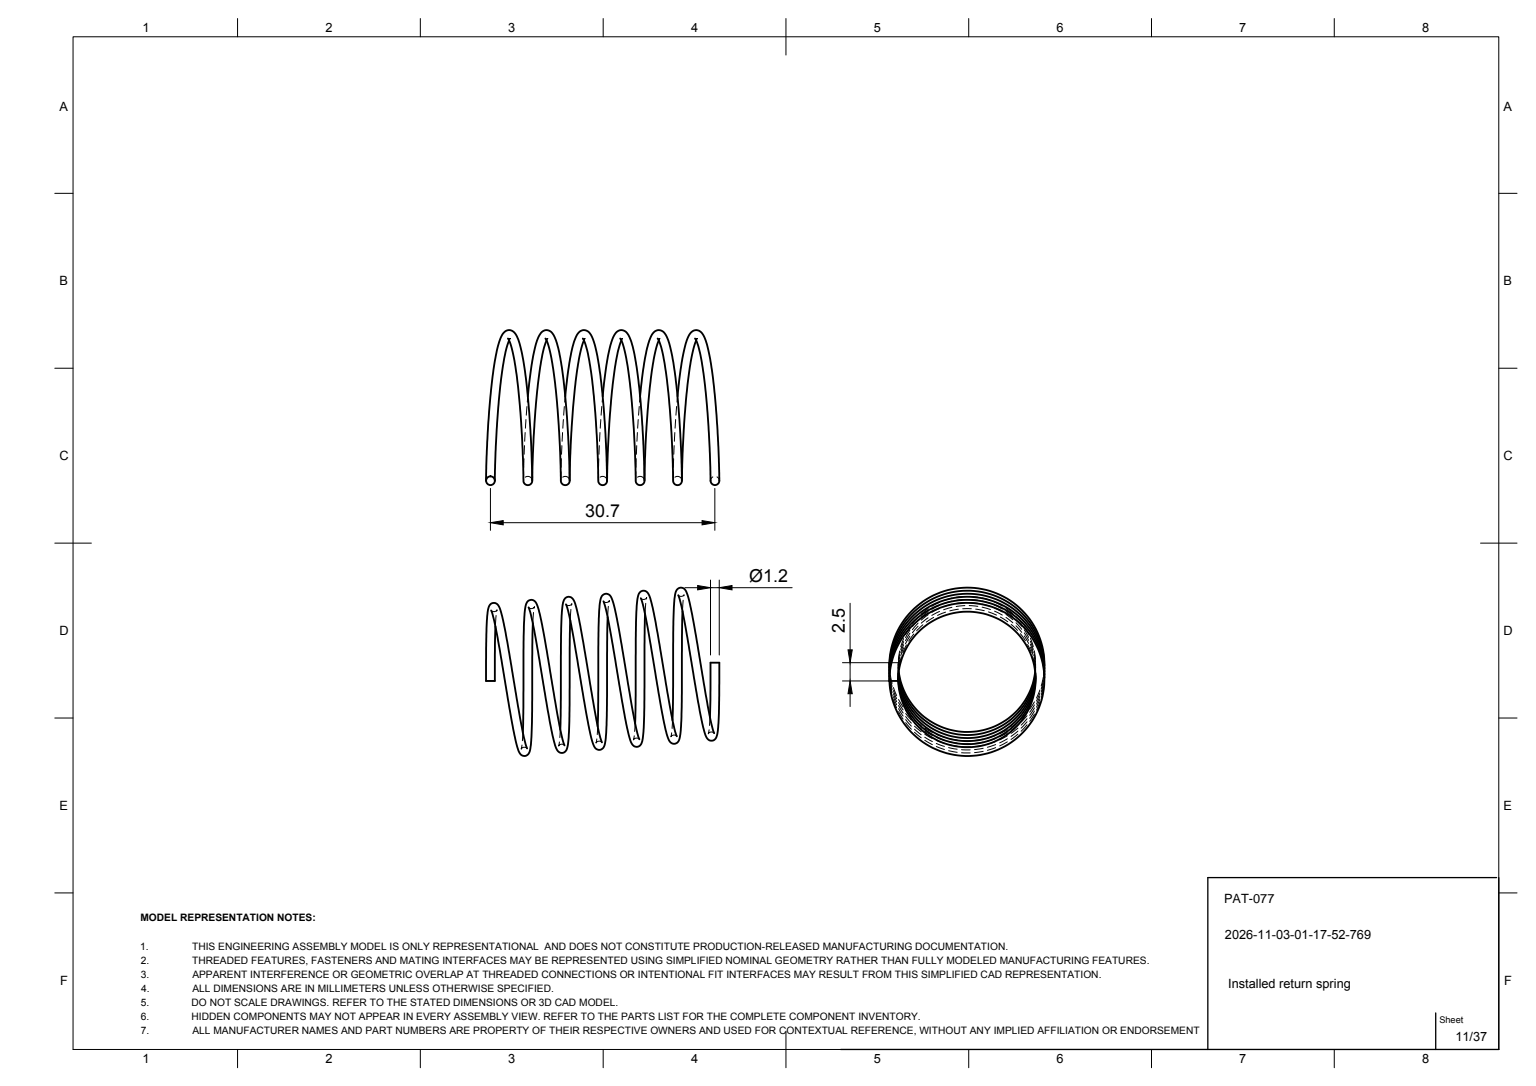
ISO-10303-21;
HEADER;
/* Generated by software containing ST-Developer
 * from STEP Tools, Inc. (www.steptools.com) 
 */

FILE_DESCRIPTION(
/* description */ ('Pallet stop with pneumatic fitting'),
/* implementation_level */ '2;1');

FILE_NAME(
/* name */ 'Installed return spring.step',
/* time_stamp */ '2026-10-27T10:51:41-07:00',
/* author */ (''),
/* organization */ (''),
/* preprocessor_version */ 'ST-DEVELOPER v20.2',
/* originating_system */ 'Autodesk Translation Framework v15.17.0.0',
/* authorisation */ '');

FILE_SCHEMA (('AUTOMOTIVE_DESIGN { 1 0 10303 214 3 1 1 }'));
ENDSEC;

DATA;
#10=MECHANICAL_DESIGN_GEOMETRIC_PRESENTATION_REPRESENTATION('',(#363),#10265);
#280=B_SPLINE_CURVE_WITH_KNOTS('',3,(#8824,#8825,#8826,#8827,#8828,#8829,
#8830,#8831,#8832,#8833,#8834,#8835,#8836,#8837,#8838,#8839,#8840,#8841,
#8842,#8843,#8844,#8845,#8846,#8847,#8848,#8849,#8850,#8851,#8852,#8853,
#8854,#8855,#8856,#8857,#8858,#8859,#8860,#8861,#8862,#8863,#8864,#8865,
#8866,#8867,#8868,#8869,#8870,#8871,#8872,#8873,#8874,#8875,#8876,#8877,
#8878,#8879,#8880,#8881,#8882,#8883,#8884,#8885,#8886,#8887,#8888,#8889,
#8890,#8891,#8892,#8893,#8894,#8895,#8896,#8897,#8898,#8899),
 .UNSPECIFIED.,.F.,.F.,(4,1,1,1,1,1,1,1,1,1,1,1,1,1,1,1,1,1,1,1,1,1,1,1,
1,1,1,1,1,1,1,1,1,1,1,1,1,1,1,1,1,1,1,1,1,1,1,1,1,1,1,1,1,1,1,1,1,1,1,1,
1,1,1,1,1,1,1,1,1,1,1,1,1,4),(0.,0.0178571428571429,0.0357142857142857,
0.0535714285714286,0.0714285714285714,0.0892857142857143,0.107142857142857,
0.125,0.127232142857143,0.129464285714286,0.133928571428571,0.138392857142857,
0.142857142857143,0.158730158730159,0.174603174603175,0.19047619047619,
0.202380952380952,0.214285714285714,0.226190476190476,0.238095238095238,
0.25,0.261904761904762,0.267857142857143,0.273809523809524,0.285714285714286,
0.297619047619048,0.30952380952381,0.321428571428571,0.333333333333333,
0.349206349206349,0.365079365079365,0.373015873015873,0.380952380952381,
0.396825396825397,0.412698412698413,0.428571428571429,0.446428571428571,
0.464285714285714,0.476190476190476,0.488095238095238,0.5,0.517857142857143,
0.535714285714286,0.553571428571429,0.571428571428571,0.589285714285714,
0.607142857142857,0.625,0.642857142857143,0.651785714285714,0.660714285714286,
0.678571428571428,0.696428571428571,0.714285714285714,0.726190476190476,
0.738095238095238,0.75,0.761904761904762,0.773809523809524,0.785714285714286,
0.797619047619047,0.809523809523809,0.821428571428571,0.833333333333333,
0.845238095238095,0.857142857142857,0.875,0.892857142857143,0.910714285714286,
0.928571428571429,0.946428571428571,0.964285714285714,0.982142857142857,
1.),.UNSPECIFIED.);
#292=B_SPLINE_SURFACE_WITH_KNOTS('',3,3,((#8061,#8062,#8063,#8064,#8065,
#8066,#8067,#8068,#8069,#8070,#8071,#8072,#8073,#8074,#8075,#8076,#8077,
#8078,#8079,#8080,#8081,#8082,#8083,#8084,#8085,#8086,#8087,#8088,#8089,
#8090,#8091,#8092,#8093,#8094,#8095,#8096,#8097,#8098,#8099,#8100,#8101,
#8102,#8103,#8104,#8105,#8106,#8107,#8108,#8109,#8110,#8111,#8112,#8113,
#8114,#8115,#8116,#8117,#8118,#8119,#8120,#8121,#8122,#8123,#8124,#8125,
#8126,#8127,#8128,#8129,#8130,#8131,#8132,#8133,#8134,#8135,#8136),(#8137,
#8138,#8139,#8140,#8141,#8142,#8143,#8144,#8145,#8146,#8147,#8148,#8149,
#8150,#8151,#8152,#8153,#8154,#8155,#8156,#8157,#8158,#8159,#8160,#8161,
#8162,#8163,#8164,#8165,#8166,#8167,#8168,#8169,#8170,#8171,#8172,#8173,
#8174,#8175,#8176,#8177,#8178,#8179,#8180,#8181,#8182,#8183,#8184,#8185,
#8186,#8187,#8188,#8189,#8190,#8191,#8192,#8193,#8194,#8195,#8196,#8197,
#8198,#8199,#8200,#8201,#8202,#8203,#8204,#8205,#8206,#8207,#8208,#8209,
#8210,#8211,#8212),(#8213,#8214,#8215,#8216,#8217,#8218,#8219,#8220,#8221,
#8222,#8223,#8224,#8225,#8226,#8227,#8228,#8229,#8230,#8231,#8232,#8233,
#8234,#8235,#8236,#8237,#8238,#8239,#8240,#8241,#8242,#8243,#8244,#8245,
#8246,#8247,#8248,#8249,#8250,#8251,#8252,#8253,#8254,#8255,#8256,#8257,
#8258,#8259,#8260,#8261,#8262,#8263,#8264,#8265,#8266,#8267,#8268,#8269,
#8270,#8271,#8272,#8273,#8274,#8275,#8276,#8277,#8278,#8279,#8280,#8281,
#8282,#8283,#8284,#8285,#8286,#8287,#8288),(#8289,#8290,#8291,#8292,#8293,
#8294,#8295,#8296,#8297,#8298,#8299,#8300,#8301,#8302,#8303,#8304,#8305,
#8306,#8307,#8308,#8309,#8310,#8311,#8312,#8313,#8314,#8315,#8316,#8317,
#8318,#8319,#8320,#8321,#8322,#8323,#8324,#8325,#8326,#8327,#8328,#8329,
#8330,#8331,#8332,#8333,#8334,#8335,#8336,#8337,#8338,#8339,#8340,#8341,
#8342,#8343,#8344,#8345,#8346,#8347,#8348,#8349,#8350,#8351,#8352,#8353,
#8354,#8355,#8356,#8357,#8358,#8359,#8360,#8361,#8362,#8363,#8364),(#8365,
#8366,#8367,#8368,#8369,#8370,#8371,#8372,#8373,#8374,#8375,#8376,#8377,
#8378,#8379,#8380,#8381,#8382,#8383,#8384,#8385,#8386,#8387,#8388,#8389,
#8390,#8391,#8392,#8393,#8394,#8395,#8396,#8397,#8398,#8399,#8400,#8401,
#8402,#8403,#8404,#8405,#8406,#8407,#8408,#8409,#8410,#8411,#8412,#8413,
#8414,#8415,#8416,#8417,#8418,#8419,#8420,#8421,#8422,#8423,#8424,#8425,
#8426,#8427,#8428,#8429,#8430,#8431,#8432,#8433,#8434,#8435,#8436,#8437,
#8438,#8439,#8440),(#8441,#8442,#8443,#8444,#8445,#8446,#8447,#8448,#8449,
#8450,#8451,#8452,#8453,#8454,#8455,#8456,#8457,#8458,#8459,#8460,#8461,
#8462,#8463,#8464,#8465,#8466,#8467,#8468,#8469,#8470,#8471,#8472,#8473,
#8474,#8475,#8476,#8477,#8478,#8479,#8480,#8481,#8482,#8483,#8484,#8485,
#8486,#8487,#8488,#8489,#8490,#8491,#8492,#8493,#8494,#8495,#8496,#8497,
#8498,#8499,#8500,#8501,#8502,#8503,#8504,#8505,#8506,#8507,#8508,#8509,
#8510,#8511,#8512,#8513,#8514,#8515,#8516),(#8517,#8518,#8519,#8520,#8521,
#8522,#8523,#8524,#8525,#8526,#8527,#8528,#8529,#8530,#8531,#8532,#8533,
#8534,#8535,#8536,#8537,#8538,#8539,#8540,#8541,#8542,#8543,#8544,#8545,
#8546,#8547,#8548,#8549,#8550,#8551,#8552,#8553,#8554,#8555,#8556,#8557,
#8558,#8559,#8560,#8561,#8562,#8563,#8564,#8565,#8566,#8567,#8568,#8569,
#8570,#8571,#8572,#8573,#8574,#8575,#8576,#8577,#8578,#8579,#8580,#8581,
#8582,#8583,#8584,#8585,#8586,#8587,#8588,#8589,#8590,#8591,#8592),(#8593,
#8594,#8595,#8596,#8597,#8598,#8599,#8600,#8601,#8602,#8603,#8604,#8605,
#8606,#8607,#8608,#8609,#8610,#8611,#8612,#8613,#8614,#8615,#8616,#8617,
#8618,#8619,#8620,#8621,#8622,#8623,#8624,#8625,#8626,#8627,#8628,#8629,
#8630,#8631,#8632,#8633,#8634,#8635,#8636,#8637,#8638,#8639,#8640,#8641,
#8642,#8643,#8644,#8645,#8646,#8647,#8648,#8649,#8650,#8651,#8652,#8653,
#8654,#8655,#8656,#8657,#8658,#8659,#8660,#8661,#8662,#8663,#8664,#8665,
#8666,#8667,#8668),(#8669,#8670,#8671,#8672,#8673,#8674,#8675,#8676,#8677,
#8678,#8679,#8680,#8681,#8682,#8683,#8684,#8685,#8686,#8687,#8688,#8689,
#8690,#8691,#8692,#8693,#8694,#8695,#8696,#8697,#8698,#8699,#8700,#8701,
#8702,#8703,#8704,#8705,#8706,#8707,#8708,#8709,#8710,#8711,#8712,#8713,
#8714,#8715,#8716,#8717,#8718,#8719,#8720,#8721,#8722,#8723,#8724,#8725,
#8726,#8727,#8728,#8729,#8730,#8731,#8732,#8733,#8734,#8735,#8736,#8737,
#8738,#8739,#8740,#8741,#8742,#8743,#8744),(#8745,#8746,#8747,#8748,#8749,
#8750,#8751,#8752,#8753,#8754,#8755,#8756,#8757,#8758,#8759,#8760,#8761,
#8762,#8763,#8764,#8765,#8766,#8767,#8768,#8769,#8770,#8771,#8772,#8773,
#8774,#8775,#8776,#8777,#8778,#8779,#8780,#8781,#8782,#8783,#8784,#8785,
#8786,#8787,#8788,#8789,#8790,#8791,#8792,#8793,#8794,#8795,#8796,#8797,
#8798,#8799,#8800,#8801,#8802,#8803,#8804,#8805,#8806,#8807,#8808,#8809,
#8810,#8811,#8812,#8813,#8814,#8815,#8816,#8817,#8818,#8819,#8820)),
 .UNSPECIFIED.,.T.,.F.,.F.,(4,1,1,1,1,1,1,4),(4,1,1,1,1,1,1,1,1,1,1,1,1,
1,1,1,1,1,1,1,1,1,1,1,1,1,1,1,1,1,1,1,1,1,1,1,1,1,1,1,1,1,1,1,1,1,1,1,1,
1,1,1,1,1,1,1,1,1,1,1,1,1,1,1,1,1,1,1,1,1,1,1,1,4),(-3.14159265358979,-2.24399475256414,
-1.34639685153848,-0.448798950512828,0.448798950512828,1.34639685153848,
2.24399475256414,3.14159265358979),(0.,0.0178571428571429,0.0357142857142857,
0.0535714285714286,0.0714285714285714,0.0892857142857143,0.107142857142857,
0.125,0.127232142857143,0.129464285714286,0.133928571428571,0.138392857142857,
0.142857142857143,0.158730158730159,0.174603174603175,0.19047619047619,
0.202380952380952,0.214285714285714,0.226190476190476,0.238095238095238,
0.25,0.261904761904762,0.267857142857143,0.273809523809524,0.285714285714286,
0.297619047619048,0.30952380952381,0.321428571428571,0.333333333333333,
0.349206349206349,0.365079365079365,0.373015873015873,0.380952380952381,
0.396825396825397,0.412698412698413,0.428571428571429,0.446428571428571,
0.464285714285714,0.476190476190476,0.488095238095238,0.5,0.517857142857143,
0.535714285714286,0.553571428571429,0.571428571428571,0.589285714285714,
0.607142857142857,0.625,0.642857142857143,0.651785714285714,0.660714285714286,
0.678571428571428,0.696428571428571,0.714285714285714,0.726190476190476,
0.738095238095238,0.75,0.761904761904762,0.773809523809524,0.785714285714286,
0.797619047619047,0.809523809523809,0.821428571428571,0.833333333333333,
0.845238095238095,0.857142857142857,0.875,0.892857142857143,0.910714285714286,
0.928571428571429,0.946428571428571,0.964285714285714,0.982142857142857,
1.),.UNSPECIFIED.);
#299=SHAPE_REPRESENTATION_RELATIONSHIP('SRR','None',#10412,#331);
#331=ADVANCED_BREP_SHAPE_REPRESENTATION('',(#395),#10236);
#363=STYLED_ITEM('',(#10655),#395);
#395=MANIFOLD_SOLID_BREP('Body1',#5051);
#587=PLANE('',#5581);
#588=PLANE('',#5582);
#810=FACE_OUTER_BOUND('',#1170,.T.);
#811=FACE_OUTER_BOUND('',#1171,.T.);
#812=FACE_OUTER_BOUND('',#1172,.T.);
#1170=EDGE_LOOP('',(#3698,#3699,#3700,#3701));
#1171=EDGE_LOOP('',(#3702));
#1172=EDGE_LOOP('',(#3703));
#2224=CIRCLE('',#5579,0.06);
#2225=CIRCLE('',#5580,0.06);
#2503=VERTEX_POINT('',#8821);
#2504=VERTEX_POINT('',#8823);
#2948=EDGE_CURVE('',#2503,#2503,#2224,.T.);
#2949=EDGE_CURVE('',#2503,#2504,#280,.T.);
#2950=EDGE_CURVE('',#2504,#2504,#2225,.T.);
#3698=ORIENTED_EDGE('',*,*,#2948,.T.);
#3699=ORIENTED_EDGE('',*,*,#2949,.T.);
#3700=ORIENTED_EDGE('',*,*,#2950,.F.);
#3701=ORIENTED_EDGE('',*,*,#2949,.F.);
#3702=ORIENTED_EDGE('',*,*,#2950,.T.);
#3703=ORIENTED_EDGE('',*,*,#2948,.F.);
#4805=ADVANCED_FACE('',(#810),#292,.T.);
#4806=ADVANCED_FACE('',(#811),#587,.T.);
#4807=ADVANCED_FACE('',(#812),#588,.F.);
#5051=CLOSED_SHELL('',(#4805,#4806,#4807));
#5578=AXIS2_PLACEMENT_3D('',#8060,#6461,#6462);
#5579=AXIS2_PLACEMENT_3D('',#8822,#6463,#6464);
#5580=AXIS2_PLACEMENT_3D('',#8900,#6465,#6466);
#5581=AXIS2_PLACEMENT_3D('',#8901,#6467,#6468);
#5582=AXIS2_PLACEMENT_3D('',#8902,#6469,#6470);
#6461=DIRECTION('axis',(0.,0.,1.));
#6462=DIRECTION('refdir',(1.,0.,0.));
#6463=DIRECTION('center_axis',(-0.000134470403067858,0.996698884077706,
0.0811869225674069));
#6464=DIRECTION('ref_axis',(1.09533965337888E-5,-0.0811869218285139,0.996698893148795));
#6465=DIRECTION('center_axis',(0.000134470245157523,0.9966988840305,0.0811869231471977));
#6466=DIRECTION('ref_axis',(-0.0717698662269105,0.0809871795599261,-0.994127840395137));
#6467=DIRECTION('center_axis',(0.000134470245157523,0.9966988840305,0.0811869231471977));
#6468=DIRECTION('ref_axis',(-0.0717698662269105,0.0809871795599261,-0.994127840395137));
#6469=DIRECTION('center_axis',(-0.000134470403067858,0.996698884077706,
0.0811869225674069));
#6470=DIRECTION('ref_axis',(1.09533965337888E-5,-0.081186921828514,0.996698893148795));
#8060=CARTESIAN_POINT('',(0.,0.,0.));
#8061=CARTESIAN_POINT('Ctrl Pts',(0.999999342796208,0.0048712153097108,
8.80019806641107));
#8062=CARTESIAN_POINT('Ctrl Pts',(0.99996896462742,0.230035163961994,8.81853897995701));
#8063=CARTESIAN_POINT('Ctrl Pts',(0.843216945008081,0.678245689353448,8.85526000727444));
#8064=CARTESIAN_POINT('Ctrl Pts',(0.23714388778331,1.05999084182087,8.91053070559157));
#8065=CARTESIAN_POINT('Ctrl Pts',(-0.476746387578999,0.979670338171269,
8.96597705173729));
#8066=CARTESIAN_POINT('Ctrl Pts',(-0.98657616663209,0.470389879273211,9.0216024298575));
#8067=CARTESIAN_POINT('Ctrl Pts',(-1.06798165663575,-0.248000588468906,
9.07740270249169));
#8068=CARTESIAN_POINT('Ctrl Pts',(-0.682243081073035,-0.862304425765768,
9.1333764236107));
#8069=CARTESIAN_POINT('Ctrl Pts',(-0.196330490445415,-1.03251494397982,
9.17314484390509));
#8070=CARTESIAN_POINT('Ctrl Pts',(0.0904960552365201,-1.02015022040365,
9.19657718102618));
#8071=CARTESIAN_POINT('Ctrl Pts',(0.204441911777542,-1.00572651008441,9.20595357869542));
#8072=CARTESIAN_POINT('Ctrl Pts',(0.343951015893895,-0.96975630344906,9.21768054548145));
#8073=CARTESIAN_POINT('Ctrl Pts',(0.501773879908335,-0.899045416054097,
9.23176320323934));
#8074=CARTESIAN_POINT('Ctrl Pts',(0.768592409823833,-0.721243151610969,
9.2578611494339));
#8075=CARTESIAN_POINT('Ctrl Pts',(1.04382114359922,-0.318042243912805,9.29602676229045));
#8076=CARTESIAN_POINT('Ctrl Pts',(1.04456490155922,0.326294295864951,9.34634267499162));
#8077=CARTESIAN_POINT('Ctrl Pts',(0.711307557250243,0.815326125223123,9.39257751006242));
#8078=CARTESIAN_POINT('Ctrl Pts',(0.234442425347365,1.04427973165066,9.43469552996756));
#8079=CARTESIAN_POINT('Ctrl Pts',(-0.242097506080382,1.04460426316974,9.47266669612882));
#8080=CARTESIAN_POINT('Ctrl Pts',(-0.672296189994615,0.837312084419627,
9.51070107270169));
#8081=CARTESIAN_POINT('Ctrl Pts',(-0.970493141256397,0.463551157181226,
9.54879683116503));
#8082=CARTESIAN_POINT('Ctrl Pts',(-1.07723336834064,-0.00342794058422688,
9.58695206272228));
#8083=CARTESIAN_POINT('Ctrl Pts',(-0.988260429843343,-0.39307851175747,
9.61879599421848));
#8084=CARTESIAN_POINT('Ctrl Pts',(-0.82093539560644,-0.658946730224756,
9.64429884892662));
#8085=CARTESIAN_POINT('Ctrl Pts',(-0.598840710302034,-0.88141322392247,
9.66981982299092));
#8086=CARTESIAN_POINT('Ctrl Pts',(-0.237756057923814,-1.05547919442497,
9.70175433946707));
#8087=CARTESIAN_POINT('Ctrl Pts',(0.243905786180905,-1.05553040152794,9.74012683420727));
#8088=CARTESIAN_POINT('Ctrl Pts',(0.678604028637572,-0.846341399380819,
9.77854812145871));
#8089=CARTESIAN_POINT('Ctrl Pts',(0.979430107833126,-0.468912235308927,
9.81701586224876));
#8090=CARTESIAN_POINT('Ctrl Pts',(1.09985901046267,0.0548445677701001,9.85980673545165));
#8091=CARTESIAN_POINT('Ctrl Pts',(0.921933505746503,0.631124795915794,9.90693599171239));
#8092=CARTESIAN_POINT('Ctrl Pts',(0.4929126040201,0.973793160670524,9.94983738646297));
#8093=CARTESIAN_POINT('Ctrl Pts',(0.0780904371091028,1.06751269479759,9.98418939216924));
#8094=CARTESIAN_POINT('Ctrl Pts',(-0.346188348797786,1.0365452542535,10.0185609429505));
#8095=CARTESIAN_POINT('Ctrl Pts',(-0.822968443953264,0.76162232341949,10.0615600576428));
#8096=CARTESIAN_POINT('Ctrl Pts',(-1.11011929233597,0.166104281872854,10.1132080400722));
#8097=CARTESIAN_POINT('Ctrl Pts',(-1.0081246602054,-0.515708350877839,10.1670522944212));
#8098=CARTESIAN_POINT('Ctrl Pts',(-0.494775946618556,-1.02970801548153,
10.2230915794475));
#8099=CARTESIAN_POINT('Ctrl Pts',(0.171330015334639,-1.10394798748412,10.2748519542969));
#8100=CARTESIAN_POINT('Ctrl Pts',(0.683814393710209,-0.85633240678914,10.3201591760856));
#8101=CARTESIAN_POINT('Ctrl Pts',(0.987375224349673,-0.475369257557772,
10.3590026286433));
#8102=CARTESIAN_POINT('Ctrl Pts',(1.11501021817459,0.0796008030233853,10.4043267361272));
#8103=CARTESIAN_POINT('Ctrl Pts',(0.894257942603671,0.712772351603783,10.4561304980607));
#8104=CARTESIAN_POINT('Ctrl Pts',(0.254526418580225,1.11465334671006,10.5144063331842));
#8105=CARTESIAN_POINT('Ctrl Pts',(-0.495386650979013,1.03000796421648,10.5726689321936));
#8106=CARTESIAN_POINT('Ctrl Pts',(-1.02902006816757,0.496451864872819,10.6309084916996));
#8107=CARTESIAN_POINT('Ctrl Pts',(-1.11329107431628,-0.25302544687232,10.6891152782939));
#8108=CARTESIAN_POINT('Ctrl Pts',(-0.712411475504087,-0.890954531307481,
10.7472796615617));
#8109=CARTESIAN_POINT('Ctrl Pts',(-0.00144545535703713,-1.13970545531556,
10.8053921361455));
#8110=CARTESIAN_POINT('Ctrl Pts',(0.589562318042014,-0.932130645422847,
10.8537681412278));
#8111=CARTESIAN_POINT('Ctrl Pts',(0.908494555547074,-0.573322783618425,
10.8924337348326));
#8112=CARTESIAN_POINT('Ctrl Pts',(1.0932000203843,-0.130460109720627,10.9310743576345));
#8113=CARTESIAN_POINT('Ctrl Pts',(1.02452819258886,0.49024714203063,10.9793255246093));
#8114=CARTESIAN_POINT('Ctrl Pts',(0.493612168598575,1.02033558321459,11.037138824411));
#8115=CARTESIAN_POINT('Ctrl Pts',(-0.166230575259128,1.09368100121347,11.0884425957329));
#8116=CARTESIAN_POINT('Ctrl Pts',(-0.673140522140151,0.84850197959383,11.1332655331794));
#8117=CARTESIAN_POINT('Ctrl Pts',(-0.973483979429893,0.47222295927322,11.1716363210045));
#8118=CARTESIAN_POINT('Ctrl Pts',(-1.08028898641827,0.00311472479435195,
11.2099559586628));
#8119=CARTESIAN_POINT('Ctrl Pts',(-0.973354083483389,-0.465125791076451,
11.2482222395404));
#8120=CARTESIAN_POINT('Ctrl Pts',(-0.674252322492463,-0.840091585392608,
11.2864330284043));
#8121=CARTESIAN_POINT('Ctrl Pts',(-0.242715089956039,-1.04789098180051,
11.3245862592493));
#8122=CARTESIAN_POINT('Ctrl Pts',(0.23542767696283,-1.04765866302507,11.3626799542613));
#8123=CARTESIAN_POINT('Ctrl Pts',(0.665536159094464,-0.840435751119737,
11.4007121983223));
#8124=CARTESIAN_POINT('Ctrl Pts',(0.962591820228485,-0.467820172164233,
11.4386811727585));
#8125=CARTESIAN_POINT('Ctrl Pts',(1.06846208937938,-0.00379118886353965,
11.47658513569));
#8126=CARTESIAN_POINT('Ctrl Pts',(0.962501175338684,0.458913289962351,11.5144224357756));
#8127=CARTESIAN_POINT('Ctrl Pts',(0.618041205754224,0.892154566858533,11.5584863515166));
#8128=CARTESIAN_POINT('Ctrl Pts',(0.00421838652791971,1.10738146763147,
11.6087289304493));
#8129=CARTESIAN_POINT('Ctrl Pts',(-0.685284502455283,0.86560690604705,11.6650903417562));
#8130=CARTESIAN_POINT('Ctrl Pts',(-1.07219887432344,0.249028474249683,11.7212863124465));
#8131=CARTESIAN_POINT('Ctrl Pts',(-0.990640181337795,-0.472396051339649,
11.7773128627812));
#8132=CARTESIAN_POINT('Ctrl Pts',(-0.478640001005609,-0.983760746265736,
11.8331676524783));
#8133=CARTESIAN_POINT('Ctrl Pts',(0.238202676882345,-1.06445286799178,11.8888462567429));
#8134=CARTESIAN_POINT('Ctrl Pts',(0.846858663881909,-0.681098479204223,
11.9443505326692));
#8135=CARTESIAN_POINT('Ctrl Pts',(1.00427568511571,-0.230977292777482,11.9812290386622));
#8136=CARTESIAN_POINT('Ctrl Pts',(1.00430619197361,-0.004859230773597,11.9996476704237));
#8137=CARTESIAN_POINT('Ctrl Pts',(0.982047384939078,0.00486879330739147,
8.80019806641107));
#8138=CARTESIAN_POINT('Ctrl Pts',(0.982017542571237,0.226061368380877,8.8182154884749));
#8139=CARTESIAN_POINT('Ctrl Pts',(0.828073759479322,0.666265246409587,8.85427793870567));
#8140=CARTESIAN_POINT('Ctrl Pts',(0.232718051648345,1.04130280902705,8.90857206776144));
#8141=CARTESIAN_POINT('Ctrl Pts',(-0.468680551990921,0.962405317361456,
8.96304474127639));
#8142=CARTESIAN_POINT('Ctrl Pts',(-0.969725556632444,0.461952106094082,
9.01770706443454));
#8143=CARTESIAN_POINT('Ctrl Pts',(-1.04978892409544,-0.24421501980538,9.07255473573053));
#8144=CARTESIAN_POINT('Ctrl Pts',(-0.670526282680969,-0.848287475569065,
9.12759197393209));
#8145=CARTESIAN_POINT('Ctrl Pts',(-0.192569344974563,-1.01574821805213,
9.16670672447678));
#8146=CARTESIAN_POINT('Ctrl Pts',(0.0896475808341612,-1.00358230969371,
9.18976208492581));
#8147=CARTESIAN_POINT('Ctrl Pts',(0.201768534269143,-0.989389860609658,
9.19898826062923));
#8148=CARTESIAN_POINT('Ctrl Pts',(0.339053092327797,-0.953994606992962,
9.21052787927458));
#8149=CARTESIAN_POINT('Ctrl Pts',(0.494377601147851,-0.884404812313703,
9.22438724394839));
#8150=CARTESIAN_POINT('Ctrl Pts',(0.757001856405022,-0.709402012144092,
9.25007419376896));
#8151=CARTESIAN_POINT('Ctrl Pts',(1.0279911029959,-0.312481730693998,9.28764301092837));
#8152=CARTESIAN_POINT('Ctrl Pts',(1.02877459893023,0.322165970926696,9.33720097094436));
#8153=CARTESIAN_POINT('Ctrl Pts',(0.700413157880328,0.804092297036147,9.38275776600637));
#8154=CARTESIAN_POINT('Ctrl Pts',(0.230301769583314,1.02983016988876,9.42427724831843));
#8155=CARTESIAN_POINT('Ctrl Pts',(-0.239683635592506,1.03017515445717,9.46172242153018));
#8156=CARTESIAN_POINT('Ctrl Pts',(-0.664163045312016,0.825661502108212,
9.49924891917935));
#8157=CARTESIAN_POINT('Ctrl Pts',(-0.958529939902563,0.456745656141783,
9.53684906905032));
#8158=CARTESIAN_POINT('Ctrl Pts',(-1.06396267414552,-0.00440524776029272,
9.5745255639511));
#8159=CARTESIAN_POINT('Ctrl Pts',(-0.976079979910487,-0.389373735213914,
9.60598297021468));
#8160=CARTESIAN_POINT('Ctrl Pts',(-0.810705582541046,-0.652150929778934,
9.63118793351945));
#8161=CARTESIAN_POINT('Ctrl Pts',(-0.591146716083035,-0.872084267774335,
9.6564168813747));
#8162=CARTESIAN_POINT('Ctrl Pts',(-0.234072078906085,-1.04424533055482,
9.68799397302578));
#8163=CARTESIAN_POINT('Ctrl Pts',(0.242500469223428,-1.04432630242473,9.72595785040098));
#8164=CARTESIAN_POINT('Ctrl Pts',(0.672838065087217,-0.83726980079961,9.7639884443319));
#8165=CARTESIAN_POINT('Ctrl Pts',(0.970815428000762,-0.463458065904377,
9.80208605881035));
#8166=CARTESIAN_POINT('Ctrl Pts',(1.09019540146654,0.0555635056652221,9.84448580287717));
#8167=CARTESIAN_POINT('Ctrl Pts',(0.913813691461406,0.627036825844031,9.89121709087636));
#8168=CARTESIAN_POINT('Ctrl Pts',(0.48811414653708,0.967138669436487,9.93378708715817));
#8169=CARTESIAN_POINT('Ctrl Pts',(0.0762229670049308,1.06020598638962,9.96789328622913));
#8170=CARTESIAN_POINT('Ctrl Pts',(-0.345222042701214,1.0294593023382,10.0020337480872));
#8171=CARTESIAN_POINT('Ctrl Pts',(-0.819095169387929,0.756280403334857,
10.044760955629));
#8172=CARTESIAN_POINT('Ctrl Pts',(-1.10479169712882,0.163970602181336,10.0961315732279));
#8173=CARTESIAN_POINT('Ctrl Pts',(-1.00334187935937,-0.514754332116599,
10.1497258011113));
#8174=CARTESIAN_POINT('Ctrl Pts',(-0.491985150485256,-1.0269135369247,10.2055489936168));
#8175=CARTESIAN_POINT('Ctrl Pts',(0.172230476805367,-1.10104324987106,10.2571555969155));
#8176=CARTESIAN_POINT('Ctrl Pts',(0.6837034079542,-0.853959036612514,10.3023689497361));
#8177=CARTESIAN_POINT('Ctrl Pts',(0.986863059949987,-0.473547176850352,
10.3411560919635));
#8178=CARTESIAN_POINT('Ctrl Pts',(1.11443827396583,0.0809655868366956,10.3864406203787));
#8179=CARTESIAN_POINT('Ctrl Pts',(0.893794220249733,0.714129022372665,10.4382345485064));
#8180=CARTESIAN_POINT('Ctrl Pts',(0.253564991089117,1.11646188695564,10.4965555791176));
#8181=CARTESIAN_POINT('Ctrl Pts',(-0.497710807257122,1.03177486246381,10.5549164707911));
#8182=CARTESIAN_POINT('Ctrl Pts',(-1.03287455412715,0.496850894811073,10.6133080838302));
#8183=CARTESIAN_POINT('Ctrl Pts',(-1.11756500239139,-0.255330318551581,
10.6717198630721));
#8184=CARTESIAN_POINT('Ctrl Pts',(-0.714971732167115,-0.896204048773918,
10.7301410140639));
#8185=CARTESIAN_POINT('Ctrl Pts',(-0.000197744427673544,-1.14640555699347,
10.7885625557949));
#8186=CARTESIAN_POINT('Ctrl Pts',(0.594542321544182,-0.937612040665249,
10.8372358480802));
#8187=CARTESIAN_POINT('Ctrl Pts',(0.915705377171634,-0.576320258708504,
10.8761680572913));
#8188=CARTESIAN_POINT('Ctrl Pts',(1.10178414791373,-0.130204417591924,10.915091761851));
#8189=CARTESIAN_POINT('Ctrl Pts',(1.03265373134923,0.495463186235901,10.9637246794375));
#8190=CARTESIAN_POINT('Ctrl Pts',(0.497145233405868,1.03028230225543,11.0220401925551));
#8191=CARTESIAN_POINT('Ctrl Pts',(-0.169012977210461,1.10441503835764,11.0738304261316));
#8192=CARTESIAN_POINT('Ctrl Pts',(-0.681133539914993,0.85674905407542,11.1191103749823));
#8193=CARTESIAN_POINT('Ctrl Pts',(-0.984721103773031,0.476446874844114,
11.1578900621551));
#8194=CARTESIAN_POINT('Ctrl Pts',(-1.092751156294,0.00206620542347027,11.1966396932756));
#8195=CARTESIAN_POINT('Ctrl Pts',(-0.98459016094734,-0.471660870020862,
11.2353514494943));
#8196=CARTESIAN_POINT('Ctrl Pts',(-0.681864802424284,-0.851204764218623,
11.2740254978417));
#8197=CARTESIAN_POINT('Ctrl Pts',(-0.244894669388729,-1.06164493769735,
11.3126574520722));
#8198=CARTESIAN_POINT('Ctrl Pts',(0.239497914027533,-1.06142946990311,11.3512480535563));
#8199=CARTESIAN_POINT('Ctrl Pts',(0.675410001418759,-0.85143262563631,11.3897909190191));
#8200=CARTESIAN_POINT('Ctrl Pts',(0.97660256231849,-0.47365645262325,11.4282852412925));
#8201=CARTESIAN_POINT('Ctrl Pts',(1.08400003731686,-0.00301072745489087,
11.4667285195545));
#8202=CARTESIAN_POINT('Ctrl Pts',(0.976502876676812,0.466470502386992,11.5051182694331));
#8203=CARTESIAN_POINT('Ctrl Pts',(0.626894863562504,0.906218485725883,11.549841630365));
#8204=CARTESIAN_POINT('Ctrl Pts',(0.00363437595233928,1.12480301808217,
11.600855774006));
#8205=CARTESIAN_POINT('Ctrl Pts',(-0.696824177011358,0.879241198259212,
11.6581097453269));
#8206=CARTESIAN_POINT('Ctrl Pts',(-1.09007389999346,0.25264708501371,11.7152189643452));
#8207=CARTESIAN_POINT('Ctrl Pts',(-1.00719470908938,-0.480789320374471,
11.7721773844949));
#8208=CARTESIAN_POINT('Ctrl Pts',(-0.486528264941766,-1.00085757657432,
11.8289789551926));
#8209=CARTESIAN_POINT('Ctrl Pts',(0.242674951053419,-1.08295512724231,11.8856179806837));
#8210=CARTESIAN_POINT('Ctrl Pts',(0.861972926357441,-0.692938107583723,
11.9420899351664));
#8211=CARTESIAN_POINT('Ctrl Pts',(1.02218081422145,-0.234837326490113,11.9796219395556));
#8212=CARTESIAN_POINT('Ctrl Pts',(1.02221185564686,-0.00475702858911594,
11.9983633184843));
#8213=CARTESIAN_POINT('Ctrl Pts',(0.946251939821601,0.00346790923095878,
8.81733686319961));
#8214=CARTESIAN_POINT('Ctrl Pts',(0.946223170149248,0.216709631387298,8.83470664203795));
#8215=CARTESIAN_POINT('Ctrl Pts',(0.797868558912845,0.640717122048251,8.86944390364538));
#8216=CARTESIAN_POINT('Ctrl Pts',(0.224685675994098,1.00171482448492,8.92171403423268));
#8217=CARTESIAN_POINT('Ctrl Pts',(-0.450094354194183,0.925721174112207,
8.97411924922092));
#8218=CARTESIAN_POINT('Ctrl Pts',(-0.931851520616104,0.444457369493084,
9.02668243919957));
#8219=CARTESIAN_POINT('Ctrl Pts',(-1.00876374936087,-0.234332975359601,
9.07940345376113));
#8220=CARTESIAN_POINT('Ctrl Pts',(-0.644280498352913,-0.814814073429451,
9.132293292668));
#8221=CARTESIAN_POINT('Ctrl Pts',(-0.185030806522485,-0.975710075967432,
9.16987780176979));
#8222=CARTESIAN_POINT('Ctrl Pts',(0.0861306964382634,-0.964020787510786,
9.19203012360292));
#8223=CARTESIAN_POINT('Ctrl Pts',(0.193859203693136,-0.950384199462588,
9.20089488110907));
#8224=CARTESIAN_POINT('Ctrl Pts',(0.325766432724325,-0.916374835785051,
9.21198266561942));
#8225=CARTESIAN_POINT('Ctrl Pts',(0.475008489408351,-0.849509651707339,
9.22529946397773));
#8226=CARTESIAN_POINT('Ctrl Pts',(0.72735253136785,-0.681355419969213,9.2499813528838));
#8227=CARTESIAN_POINT('Ctrl Pts',(0.987759532431315,-0.299937694770344,
9.28608546277695));
#8228=CARTESIAN_POINT('Ctrl Pts',(0.988529254394412,0.31002344397511,9.33371680705976));
#8229=CARTESIAN_POINT('Ctrl Pts',(0.67286673528341,0.773354286803788,9.37751699303838));
#8230=CARTESIAN_POINT('Ctrl Pts',(0.220764282478621,0.990462726141864,9.41744839941452));
#8231=CARTESIAN_POINT('Ctrl Pts',(-0.23137446087799,0.990807495240239,9.45347433529735));
#8232=CARTESIAN_POINT('Ctrl Pts',(-0.639893401702073,0.794007818769354,
9.48958994897445));
#8233=CARTESIAN_POINT('Ctrl Pts',(-0.923327263108843,0.438822435846309,
9.52579447470907));
#8234=CARTESIAN_POINT('Ctrl Pts',(-1.02491137571836,-0.00538407263128216,
9.56208933392858));
#8235=CARTESIAN_POINT('Ctrl Pts',(-0.940232267608687,-0.376417877351174,
9.59241037531266));
#8236=CARTESIAN_POINT('Ctrl Pts',(-0.780786057662726,-0.629783667326523,
9.61671320097693));
#8237=CARTESIAN_POINT('Ctrl Pts',(-0.569033793255791,-0.841902767826415,
9.64104641368153));
#8238=CARTESIAN_POINT('Ctrl Pts',(-0.224489149210013,-1.0080482857871,9.67151952337384));
#8239=CARTESIAN_POINT('Ctrl Pts',(0.235673510791263,-1.00815805640934,9.70817893472068));
#8240=CARTESIAN_POINT('Ctrl Pts',(0.651503567024935,-0.808120949371662,
9.74492970282906));
#8241=CARTESIAN_POINT('Ctrl Pts',(0.939670159494493,-0.446677535335527,
9.78177187806484));
#8242=CARTESIAN_POINT('Ctrl Pts',(1.05523972468657,0.0555890051172364,9.82280879182749));
#8243=CARTESIAN_POINT('Ctrl Pts',(0.884483903066246,0.609188073050605,9.86807884630888));
#8244=CARTESIAN_POINT('Ctrl Pts',(0.471693669376953,0.939087262360839,9.90936701071719));
#8245=CARTESIAN_POINT('Ctrl Pts',(0.0718701946233878,1.02945078127861,9.94247676831493));
#8246=CARTESIAN_POINT('Ctrl Pts',(-0.337475699762535,0.999603452125411,
9.97563909649433));
#8247=CARTESIAN_POINT('Ctrl Pts',(-0.798276925818471,0.734084817620259,
10.0171900420759));
#8248=CARTESIAN_POINT('Ctrl Pts',(-1.0765334634925,0.157487645860965,10.0672053034725));
#8249=CARTESIAN_POINT('Ctrl Pts',(-0.977769536461385,-0.504250043799724,
10.1194626321329));
#8250=CARTESIAN_POINT('Ctrl Pts',(-0.478575291848728,-1.00451835916292,
10.1739816819444));
#8251=CARTESIAN_POINT('Ctrl Pts',(0.171126569807208,-1.07721754138009,10.2244700816925));
#8252=CARTESIAN_POINT('Ctrl Pts',(0.672182788674072,-0.835256219302107,
10.2687619732111));
#8253=CARTESIAN_POINT('Ctrl Pts',(0.969547810320499,-0.462213248235356,
10.3068036909456));
#8254=CARTESIAN_POINT('Ctrl Pts',(1.09489348151214,0.0822563931149444,10.3512740281145));
#8255=CARTESIAN_POINT('Ctrl Pts',(0.878086601000876,0.705028239333339,10.4022206349257));
#8256=CARTESIAN_POINT('Ctrl Pts',(0.247376731962901,1.10167051144662,10.4596936844876));
#8257=CARTESIAN_POINT('Ctrl Pts',(-0.494343825650103,1.01831274777828,10.5173179494214));
#8258=CARTESIAN_POINT('Ctrl Pts',(-1.02389367392556,0.489356402466505,10.5750854103097));
#8259=CARTESIAN_POINT('Ctrl Pts',(-1.1080879323535,-0.256139394666961,10.6329877640774));
#8260=CARTESIAN_POINT('Ctrl Pts',(-0.708467620348485,-0.892752715736136,
10.6910165384584));
#8261=CARTESIAN_POINT('Ctrl Pts',(0.00275806339120792,-1.14199252167361,
10.7491621240617));
#8262=CARTESIAN_POINT('Ctrl Pts',(0.595915072591307,-0.933982364866608,
10.7977073894074));
#8263=CARTESIAN_POINT('Ctrl Pts',(0.916693997947134,-0.573186172446775,
10.8365910184109));
#8264=CARTESIAN_POINT('Ctrl Pts',(1.10275571560074,-0.127229568265828,10.8755054547366));
#8265=CARTESIAN_POINT('Ctrl Pts',(1.03374107847987,0.499230126741185,10.9242044521008));
#8266=CARTESIAN_POINT('Ctrl Pts',(0.496651096330989,1.03602339561547,10.982721896355));
#8267=CARTESIAN_POINT('Ctrl Pts',(-0.173057151953294,1.11077134701646,11.0347972056812));
#8268=CARTESIAN_POINT('Ctrl Pts',(-0.688810280773869,0.861454433490338,
11.0803977479046));
#8269=CARTESIAN_POINT('Ctrl Pts',(-0.994990321540318,0.478015999913525,
11.1195067251792));
#8270=CARTESIAN_POINT('Ctrl Pts',(-1.10413900699883,-0.000930907827253689,
11.1586323799395));
#8271=CARTESIAN_POINT('Ctrl Pts',(-0.994852434030972,-0.479892724154501,
11.1977747838273));
#8272=CARTESIAN_POINT('Ctrl Pts',(-0.688454851688791,-0.864158828181502,
11.2369285531699));
#8273=CARTESIAN_POINT('Ctrl Pts',(-0.245556936433115,-1.07753293814173,
11.2760917573129));
#8274=CARTESIAN_POINT('Ctrl Pts',(0.246044401600366,-1.0773877681717,11.3152583014517));
#8275=CARTESIAN_POINT('Ctrl Pts',(0.689038817571119,-0.864056889518542,
11.3544280678403));
#8276=CARTESIAN_POINT('Ctrl Pts',(0.995533503363568,-0.479743995432174,
11.3935962007367));
#8277=CARTESIAN_POINT('Ctrl Pts',(1.10500493611492,-0.000336441793609564,
11.432759423983));
#8278=CARTESIAN_POINT('Ctrl Pts',(0.995437508199075,0.478484225555593,11.471914533027));
#8279=CARTESIAN_POINT('Ctrl Pts',(0.638543403370204,0.927530552036555,11.5175815981191));
#8280=CARTESIAN_POINT('Ctrl Pts',(0.00131834384992748,1.1512205599446,11.5697498749575));
#8281=CARTESIAN_POINT('Ctrl Pts',(-0.716162033397229,0.899924142153474,
11.6283938640621));
#8282=CARTESIAN_POINT('Ctrl Pts',(-1.11974363778359,0.257254170951805,11.6869825988179));
#8283=CARTESIAN_POINT('Ctrl Pts',(-1.03478697806096,-0.496287761111256,
11.7455056502723));
#8284=CARTESIAN_POINT('Ctrl Pts',(-0.499211397844794,-1.0315157806068,11.8039508889109));
#8285=CARTESIAN_POINT('Ctrl Pts',(0.25207649193241,-1.11624858861966,11.8623120440781));
#8286=CARTESIAN_POINT('Ctrl Pts',(0.891057567372483,-0.71406944827229,11.9205699244295));
#8287=CARTESIAN_POINT('Ctrl Pts',(1.05664899061948,-0.24083687143616,11.9593476619553));
#8288=CARTESIAN_POINT('Ctrl Pts',(1.05668105685756,-0.00316062068079096,
11.9787077754391));
#8289=CARTESIAN_POINT('Ctrl Pts',(0.933110845774544,-0.00124761587970791,
8.87520568466563));
#8290=CARTESIAN_POINT('Ctrl Pts',(0.933082485311987,0.208961030315505,8.89232840182152));
#8291=CARTESIAN_POINT('Ctrl Pts',(0.786770179169481,0.626345163412827,8.92653493659135));
#8292=CARTESIAN_POINT('Ctrl Pts',(0.224133602875593,0.980245228608542,8.97782692366071));
#8293=CARTESIAN_POINT('Ctrl Pts',(-0.435812671372105,0.905573247736591,
9.02908909375654));
#8294=CARTESIAN_POINT('Ctrl Pts',(-0.905278949446739,0.436102668627462,
9.08034196302577));
#8295=CARTESIAN_POINT('Ctrl Pts',(-0.979701853601785,-0.223724459540056,
9.13159318793611));
#8296=CARTESIAN_POINT('Ctrl Pts',(-0.626199332431556,-0.786111248844846,
9.18285439354528));
#8297=CARTESIAN_POINT('Ctrl Pts',(-0.182309307756624,-0.941401852206475,
9.21918157669349));
#8298=CARTESIAN_POINT('Ctrl Pts',(0.0793196104033138,-0.930122621318997,
9.24055595057928));
#8299=CARTESIAN_POINT('Ctrl Pts',(0.183226682424838,-0.916969037284389,
9.24910628913725));
#8300=CARTESIAN_POINT('Ctrl Pts',(0.310391085781095,-0.884178026616486,
9.25979589713383));
#8301=CARTESIAN_POINT('Ctrl Pts',(0.454169054244644,-0.819756142740368,
9.27262568518493));
#8302=CARTESIAN_POINT('Ctrl Pts',(0.697116053142912,-0.657850695056992,
9.29638934987471));
#8303=CARTESIAN_POINT('Ctrl Pts',(0.947351969011777,-0.291063703435681,
9.33110485588488));
#8304=CARTESIAN_POINT('Ctrl Pts',(0.947893979854482,0.294038239775498,9.37679585569485));
#8305=CARTESIAN_POINT('Ctrl Pts',(0.64559614597452,0.737470402080906,9.41872694647258));
#8306=CARTESIAN_POINT('Ctrl Pts',(0.213542771693588,0.944865687214638,9.456887453317));
#8307=CARTESIAN_POINT('Ctrl Pts',(-0.21790942255983,0.945130416632738,9.49126781446859));
#8308=CARTESIAN_POINT('Ctrl Pts',(-0.607175295083612,0.757538118255783,
9.52568490650978));
#8309=CARTESIAN_POINT('Ctrl Pts',(-0.876886139203015,0.419454940311435,
9.5601447217719));
#8310=CARTESIAN_POINT('Ctrl Pts',(-0.973399204055829,-0.00281983355499825,
9.59464850829951));
#8311=CARTESIAN_POINT('Ctrl Pts',(-0.892953621384232,-0.355121345095021,
9.62344157007163));
#8312=CARTESIAN_POINT('Ctrl Pts',(-0.741670531971874,-0.595502068510008,
9.64649995731916));
#8313=CARTESIAN_POINT('Ctrl Pts',(-0.540861334347598,-0.79664831552706,
9.66957548515654));
#8314=CARTESIAN_POINT('Ctrl Pts',(-0.214347909139945,-0.954058224911974,
9.69845416164799));
#8315=CARTESIAN_POINT('Ctrl Pts',(0.221317761541613,-0.954121235060302,
9.73316338989386));
#8316=CARTESIAN_POINT('Ctrl Pts',(0.614674372570484,-0.764854624133257,
9.76793103575109));
#8317=CARTESIAN_POINT('Ctrl Pts',(0.887052993147029,-0.423164929085746,
9.80275900129157));
#8318=CARTESIAN_POINT('Ctrl Pts',(0.996196176963173,0.0513246907769201,
9.8415273466477));
#8319=CARTESIAN_POINT('Ctrl Pts',(0.834948113879409,0.573926065074171,9.88426514494727));
#8320=CARTESIAN_POINT('Ctrl Pts',(0.44547575217633,0.885137394010584,9.92321920683063));
#8321=CARTESIAN_POINT('Ctrl Pts',(0.0684014908627373,0.970356094387837,
9.95444592358018));
#8322=CARTESIAN_POINT('Ctrl Pts',(-0.317575790754665,0.942207118119873,
9.98571530594194));
#8323=CARTESIAN_POINT('Ctrl Pts',(-0.751956369176069,0.691895051315754,
10.0248858146619));
#8324=CARTESIAN_POINT('Ctrl Pts',(-1.01420012669963,0.148454419987656,10.0720248209112));
#8325=CARTESIAN_POINT('Ctrl Pts',(-0.921125606711717,-0.475192219958838,
10.1212746978924));
#8326=CARTESIAN_POINT('Ctrl Pts',(-0.450640791192364,-0.946727050507445,
10.1726608327701));
#8327=CARTESIAN_POINT('Ctrl Pts',(0.161885358038663,-1.0153085919114,10.2202607279042));
#8328=CARTESIAN_POINT('Ctrl Pts',(0.634464325836929,-0.7871254203658,10.2620342877094));
#8329=CARTESIAN_POINT('Ctrl Pts',(0.915044949089008,-0.435171331085412,
10.2979265084477));
#8330=CARTESIAN_POINT('Ctrl Pts',(1.0333921730293,0.0787559345129345,10.3399027505605));
#8331=CARTESIAN_POINT('Ctrl Pts',(0.828697304223945,0.667017539209564,10.3880228606081));
#8332=CARTESIAN_POINT('Ctrl Pts',(0.232467374207285,1.04212743993356,10.4423591262489));
#8333=CARTESIAN_POINT('Ctrl Pts',(-0.469582947467488,0.963374254330498,
10.4968986206485));
#8334=CARTESIAN_POINT('Ctrl Pts',(-0.971549690422633,0.462203568299623,
10.5516426651414));
#8335=CARTESIAN_POINT('Ctrl Pts',(-1.05163594424887,-0.245277711367363,
10.6065920927203));
#8336=CARTESIAN_POINT('Ctrl Pts',(-0.671962136426674,-0.850494803107478,
10.6617469196619));
#8337=CARTESIAN_POINT('Ctrl Pts',(0.00514473529517556,-1.08801203030429,
10.7171069354582));
#8338=CARTESIAN_POINT('Ctrl Pts',(0.571006381985689,-0.889777195779423,
10.7634098332665));
#8339=CARTESIAN_POINT('Ctrl Pts',(0.877482655626295,-0.545130724676744,
10.8005540126445));
#8340=CARTESIAN_POINT('Ctrl Pts',(1.05543893274011,-0.118705473665279,10.8377653530311));
#8341=CARTESIAN_POINT('Ctrl Pts',(0.989557126951709,0.481292167662269,10.8844038712234));
#8342=CARTESIAN_POINT('Ctrl Pts',(0.474249124300982,0.996731925119642,10.9405665516539));
#8343=CARTESIAN_POINT('Ctrl Pts',(-0.170018784224988,1.06889843758203,10.9906607188205));
#8344=CARTESIAN_POINT('Ctrl Pts',(-0.667252349418254,0.828652140244528,
11.0346171254776));
#8345=CARTESIAN_POINT('Ctrl Pts',(-0.962957118749545,0.458476875796659,
11.0723761453514));
#8346=CARTESIAN_POINT('Ctrl Pts',(-1.06861617984619,-0.00474659541608284,
11.1102178529854));
#8347=CARTESIAN_POINT('Ctrl Pts',(-0.962829285747689,-0.468812774742328,
11.1481382421668));
#8348=CARTESIAN_POINT('Ctrl Pts',(-0.66552637265583,-0.841826091853817,
11.1861371971565));
#8349=CARTESIAN_POINT('Ctrl Pts',(-0.234945846970159,-1.0493782184629,11.2242118409212));
#8350=CARTESIAN_POINT('Ctrl Pts',(0.243922228184406,-1.04933364959166,11.2623624755123));
#8351=CARTESIAN_POINT('Ctrl Pts',(0.676275279337915,-0.841241205435662,
11.3005845553303));
#8352=CARTESIAN_POINT('Ctrl Pts',(0.976019367363091,-0.465554703444286,
11.3388772265428));
#8353=CARTESIAN_POINT('Ctrl Pts',(1.08335811630658,0.00404254183906937,
11.3772382701768));
#8354=CARTESIAN_POINT('Ctrl Pts',(0.975916530883124,0.474019295230167,11.4156652984567));
#8355=CARTESIAN_POINT('Ctrl Pts',(0.625055282289429,0.915683137019696,11.4605716003999));
#8356=CARTESIAN_POINT('Ctrl Pts',(-0.00300719915789507,1.13650050171769,
11.5119933522144));
#8357=CARTESIAN_POINT('Ctrl Pts',(-0.712553859124697,0.888397715677925,
11.5699732202525));
#8358=CARTESIAN_POINT('Ctrl Pts',(-1.1131339679836,0.251233314201274,11.6280728566751));
#8359=CARTESIAN_POINT('Ctrl Pts',(-1.02901641656587,-0.498400062976102,
11.6862845413367));
#8360=CARTESIAN_POINT('Ctrl Pts',(-0.494901381262588,-1.03273028842869,
11.7445959726463));
#8361=CARTESIAN_POINT('Ctrl Pts',(0.256963427041344,-1.11790522486644,11.8030028921807));
#8362=CARTESIAN_POINT('Ctrl Pts',(0.898645546609871,-0.714501447365378,
11.8614828340231));
#8363=CARTESIAN_POINT('Ctrl Pts',(1.06558957851034,-0.237981063051787,11.900531417317));
#8364=CARTESIAN_POINT('Ctrl Pts',(1.0656219039434,0.00161635137504347,11.9200480207597));
#8365=CARTESIAN_POINT('Ctrl Pts',(0.970174595120126,-0.00503563731106881,
8.92177107464792));
#8366=CARTESIAN_POINT('Ctrl Pts',(0.97014513332141,0.213336147360704,8.93955872692312));
#8367=CARTESIAN_POINT('Ctrl Pts',(0.818084749800134,0.646712210522538,8.97507667223915));
#8368=CARTESIAN_POINT('Ctrl Pts',(0.235394562966291,1.01281040837635,9.02817474980784));
#8369=CARTESIAN_POINT('Ctrl Pts',(-0.445899628158482,0.93542064652562,9.08109684256912));
#8370=CARTESIAN_POINT('Ctrl Pts',(-0.92891112461198,0.451907699888587,9.13385094731592));
#8371=CARTESIAN_POINT('Ctrl Pts',(-1.00493384222522,-0.225268939789807,
9.18644257275678));
#8372=CARTESIAN_POINT('Ctrl Pts',(-0.642976055403776,-0.800405537674571,
9.23888044258555));
#8373=CARTESIAN_POINT('Ctrl Pts',(-0.190252948988789,-0.958506313741143,
9.27591831988632));
#8374=CARTESIAN_POINT('Ctrl Pts',(0.0760513139059781,-0.947021503110477,
9.29767447763811));
#8375=CARTESIAN_POINT('Ctrl Pts',(0.181774589175,-0.933637477829087,9.30637415940269));
#8376=CARTESIAN_POINT('Ctrl Pts',(0.311077731563098,-0.900290110612741,
9.31724319560765));
#8377=CARTESIAN_POINT('Ctrl Pts',(0.457151798821983,-0.834835030372344,
9.33027774261818));
#8378=CARTESIAN_POINT('Ctrl Pts',(0.703776523677854,-0.670467504751259,
9.35440044234417));
#8379=CARTESIAN_POINT('Ctrl Pts',(0.957142808831923,-0.298758897479058,
9.38956627149585));
#8380=CARTESIAN_POINT('Ctrl Pts',(0.957424510406942,0.292287109831173,9.43571919831589));
#8381=CARTESIAN_POINT('Ctrl Pts',(0.652789107737886,0.738706737228365,9.47794167639263));
#8382=CARTESIAN_POINT('Ctrl Pts',(0.218804460523358,0.946882426971243,9.51626539400664));
#8383=CARTESIAN_POINT('Ctrl Pts',(-0.213532779418316,0.947038202528517,
9.55071209496058));
#8384=CARTESIAN_POINT('Ctrl Pts',(-0.602655482246472,0.759384664282859,
9.58511969001727));
#8385=CARTESIAN_POINT('Ctrl Pts',(-0.871589920010413,0.42210069020356,9.61948765332899));
#8386=CARTESIAN_POINT('Ctrl Pts',(-0.967523567997481,0.00184733610570532,
9.653821175649));
#8387=CARTESIAN_POINT('Ctrl Pts',(-0.887562212018797,-0.347914027050768,
9.68240518610407));
#8388=CARTESIAN_POINT('Ctrl Pts',(-0.737597515612331,-0.586165380726041,
9.70525951581694));
#8389=CARTESIAN_POINT('Ctrl Pts',(-0.538767917261371,-0.785303060437251,
9.72810483743237));
#8390=CARTESIAN_POINT('Ctrl Pts',(-0.216019756644109,-0.940798544572053,
9.75664373683193));
#8391=CARTESIAN_POINT('Ctrl Pts',(0.213607429628279,-0.940753217150432,
9.7908691867679));
#8392=CARTESIAN_POINT('Ctrl Pts',(0.60059962902176,-0.754427589325977,9.8250751579334));
#8393=CARTESIAN_POINT('Ctrl Pts',(0.867933207756893,-0.418899848761693,
9.85926601803759));
#8394=CARTESIAN_POINT('Ctrl Pts',(0.974739488850976,0.0459663586074821,
9.89724109276077));
#8395=CARTESIAN_POINT('Ctrl Pts',(0.816946688402954,0.556586882372049,9.93900235474234));
#8396=CARTESIAN_POINT('Ctrl Pts',(0.43728553409625,0.859707800736691,9.97695998576935));
#8397=CARTESIAN_POINT('Ctrl Pts',(0.0705800023320674,0.9425400029561,10.0073260394253));
#8398=CARTESIAN_POINT('Ctrl Pts',(-0.304294465461892,0.915163773381358,
10.0376942387437));
#8399=CARTESIAN_POINT('Ctrl Pts',(-0.725224446706966,0.672378460587817,
10.0756555841161));
#8400=CARTESIAN_POINT('Ctrl Pts',(-0.978574572485742,0.146870510254935,
10.1212292346273));
#8401=CARTESIAN_POINT('Ctrl Pts',(-0.888584387525938,-0.454575686059261,
10.1687245791249));
#8402=CARTESIAN_POINT('Ctrl Pts',(-0.435769223197817,-0.907990577502227,
10.2181541230081));
#8403=CARTESIAN_POINT('Ctrl Pts',(0.152021146808637,-0.973556519824532,
10.263825841961));
#8404=CARTESIAN_POINT('Ctrl Pts',(0.604566615086981,-0.754940950053836,
10.3038313663868));
#8405=CARTESIAN_POINT('Ctrl Pts',(0.872819826465687,-0.418341246999725,
10.3381524858387));
#8406=CARTESIAN_POINT('Ctrl Pts',(0.985741421500406,0.0724135376997006,
10.3782322375385));
#8407=CARTESIAN_POINT('Ctrl Pts',(0.790438866129083,0.633079182429389,10.4240968327084));
#8408=CARTESIAN_POINT('Ctrl Pts',(0.223085878751149,0.989766778797461,10.475788493229));
#8409=CARTESIAN_POINT('Ctrl Pts',(-0.443636411700346,0.91478193674211,10.527582683884));
#8410=CARTESIAN_POINT('Ctrl Pts',(-0.919485443943618,0.43944156877107,10.5794894871194));
#8411=CARTESIAN_POINT('Ctrl Pts',(-0.995164253076116,-0.230475400336733,
10.6315180175327));
#8412=CARTESIAN_POINT('Ctrl Pts',(-0.635988207832033,-0.802768774991268,
10.6836769758179));
#8413=CARTESIAN_POINT('Ctrl Pts',(0.00372743422999969,-1.02704830689769,
10.7359754361821));
#8414=CARTESIAN_POINT('Ctrl Pts',(0.537816073043853,-0.839863792888686,
10.7796792126973));
#8415=CARTESIAN_POINT('Ctrl Pts',(0.826941185002114,-0.51471177031735,10.8147214066431));
#8416=CARTESIAN_POINT('Ctrl Pts',(0.994767696821434,-0.11252633051923,10.8498165152454));
#8417=CARTESIAN_POINT('Ctrl Pts',(0.932614102397896,0.453135513169429,10.893785840357));
#8418=CARTESIAN_POINT('Ctrl Pts',(0.446931472105046,0.938895669176947,10.9467167749459));
#8419=CARTESIAN_POINT('Ctrl Pts',(-0.160185357817544,1.00689283818422,10.9939220689488));
#8420=CARTESIAN_POINT('Ctrl Pts',(-0.62876276007964,0.780495118745785,11.0353450150309));
#8421=CARTESIAN_POINT('Ctrl Pts',(-0.907457292336147,0.431620682347231,
11.0709316429417));
#8422=CARTESIAN_POINT('Ctrl Pts',(-1.00706550093635,-0.00502807237038878,
11.1066026010044));
#8423=CARTESIAN_POINT('Ctrl Pts',(-0.907333018059293,-0.442590496284849,
11.1423573938483));
#8424=CARTESIAN_POINT('Ctrl Pts',(-0.626930395137068,-0.794427236840942,
11.1781982571942));
#8425=CARTESIAN_POINT('Ctrl Pts',(-0.220647298824694,-0.990289626669596,
11.2141257343577));
#8426=CARTESIAN_POINT('Ctrl Pts',(0.231426710381895,-0.990273776039337,
11.2501419138969));
#8427=CARTESIAN_POINT('Ctrl Pts',(0.639831749928173,-0.793739088548,11.2862464373884));
#8428=CARTESIAN_POINT('Ctrl Pts',(0.923168828792549,-0.43866823784993,11.3224405845602));
#8429=CARTESIAN_POINT('Ctrl Pts',(1.0247318209223,0.0054897969252295,11.3587249749106));
#8430=CARTESIAN_POINT('Ctrl Pts',(0.923067333024604,0.450369874564741,11.3951000868224));
#8431=CARTESIAN_POINT('Ctrl Pts',(0.590716128822805,0.868819753923387,11.4376441375946));
#8432=CARTESIAN_POINT('Ctrl Pts',(-0.00492338137778625,1.0783947024351,
11.4864178746861));
#8433=CARTESIAN_POINT('Ctrl Pts',(-0.678977034279962,0.842905562412496,
11.5414947246563));
#8434=CARTESIAN_POINT('Ctrl Pts',(-1.06028826449987,0.236776613170064,11.5967771211505));
#8435=CARTESIAN_POINT('Ctrl Pts',(-0.980329318877891,-0.477775118277444,
11.6522652599988));
#8436=CARTESIAN_POINT('Ctrl Pts',(-0.470413594001006,-0.988225256329599,
11.7079556521475));
#8437=CARTESIAN_POINT('Ctrl Pts',(0.249062373267229,-1.06999291276201,11.7638509027688));
#8438=CARTESIAN_POINT('Ctrl Pts',(0.864611352792192,-0.683332131784587,
11.8199382283231));
#8439=CARTESIAN_POINT('Ctrl Pts',(1.02527007578566,-0.225384236483218,11.8574728609456));
#8440=CARTESIAN_POINT('Ctrl Pts',(1.02530118372115,0.00518903684214906,
11.8762543955908));
#8441=CARTESIAN_POINT('Ctrl Pts',(1.02975721923246,-0.00501326104248905,
8.92159505735362));
#8442=CARTESIAN_POINT('Ctrl Pts',(1.02972597594797,0.226562952611486,8.94045828718835));
#8443=CARTESIAN_POINT('Ctrl Pts',(0.86837094344991,0.686546493545894,8.97815772733461));
#8444=CARTESIAN_POINT('Ctrl Pts',(0.25006196000382,1.0749630458525,9.03449802178365));
#8445=CARTESIAN_POINT('Ctrl Pts',(-0.472771913624819,0.992854014976237,
9.09065090430009));
#8446=CARTESIAN_POINT('Ctrl Pts',(-0.985019752728312,0.479982040438132,
9.14660306370138));
#8447=CARTESIAN_POINT('Ctrl Pts',(-1.06552888416002,-0.237875691236344,
9.2023562706398));
#8448=CARTESIAN_POINT('Ctrl Pts',(-0.682010172306705,-0.847083596841777,
9.25790631176331));
#8449=CARTESIAN_POINT('Ctrl Pts',(-0.202814134616569,-1.01433803010485,
9.29710989140601));
#8450=CARTESIAN_POINT('Ctrl Pts',(0.0788679011663583,-1.00218874924703,
9.32012268492401));
#8451=CARTESIAN_POINT('Ctrl Pts',(0.190681245832686,-0.988033404006502,
9.32932353240439));
#8452=CARTESIAN_POINT('Ctrl Pts',(0.327404814279713,-0.952769801991741,
9.34081658256902));
#8453=CARTESIAN_POINT('Ctrl Pts',(0.481815903298182,-0.883576107595531,
9.35459540007272));
#8454=CARTESIAN_POINT('Ctrl Pts',(0.742439859809724,-0.709871646472506,
9.38008794825078));
#8455=CARTESIAN_POINT('Ctrl Pts',(1.00993756139607,-0.317273228204009,9.417228448983));
#8456=CARTESIAN_POINT('Ctrl Pts',(1.0101057984205,0.30611713919737,9.46590779494714));
#8457=CARTESIAN_POINT('Ctrl Pts',(0.68913686078465,0.776249633888103,9.51038260407111));
#8458=CARTESIAN_POINT('Ctrl Pts',(0.232608623129516,0.995159965668924,9.55069684565993));
#8459=CARTESIAN_POINT('Ctrl Pts',(-0.221612783036091,0.995256986950812,
9.58688996014151));
#8460=CARTESIAN_POINT('Ctrl Pts',(-0.629867340389913,0.798302867057984,
9.62299299529222));
#8461=CARTESIAN_POINT('Ctrl Pts',(-0.911611061773582,0.444834495495162,
9.65900815200399));
#8462=CARTESIAN_POINT('Ctrl Pts',(-1.01191808941633,0.00508561341048963,
9.69493535750616));
#8463=CARTESIAN_POINT('Ctrl Pts',(-0.928311649430149,-0.360330144567805,
9.72480279674522));
#8464=CARTESIAN_POINT('Ctrl Pts',(-0.771806399654962,-0.608946941831366,
9.74865322870009));
#8465=CARTESIAN_POINT('Ctrl Pts',(-0.56447207066945,-0.81658281100874,9.77247530670478));
#8466=CARTESIAN_POINT('Ctrl Pts',(-0.228304054980772,-0.97846315009502,
9.80220116775789));
#8467=CARTESIAN_POINT('Ctrl Pts',(0.218386224671673,-0.97832648895643,9.83778856842642));
#8468=CARTESIAN_POINT('Ctrl Pts',(0.62000742826206,-0.784853582088767,9.87329465940624));
#8469=CARTESIAN_POINT('Ctrl Pts',(0.896904593067191,-0.437180626270341,
9.90872029217887));
#8470=CARTESIAN_POINT('Ctrl Pts',(1.00724607137228,0.0435831230782877,9.94799570611922));
#8471=CARTESIAN_POINT('Ctrl Pts',(0.844239597184889,0.57038071251276,9.99108817060923));
#8472=CARTESIAN_POINT('Ctrl Pts',(0.453398116619752,0.882165967328861,10.0301536130233));
#8473=CARTESIAN_POINT('Ctrl Pts',(0.0767926029015151,0.96719411053426,10.0613423168352));
#8474=CARTESIAN_POINT('Ctrl Pts',(-0.307678099377883,0.939075809396451,
10.0924888336935));
#8475=CARTESIAN_POINT('Ctrl Pts',(-0.738398945185493,0.690405637103079,
10.1313486661221));
#8476=CARTESIAN_POINT('Ctrl Pts',(-0.996717094215216,0.153989961224338,
10.1778602455462));
#8477=CARTESIAN_POINT('Ctrl Pts',(-0.904871139950366,-0.457998784943317,
10.2261955249004));
#8478=CARTESIAN_POINT('Ctrl Pts',(-0.445258050472082,-0.917694255083475,
10.2763447701295));
#8479=CARTESIAN_POINT('Ctrl Pts',(0.149034788405817,-0.983646387217854,
10.3225265250447));
#8480=CARTESIAN_POINT('Ctrl Pts',(0.605170989433338,-0.76314561160354,10.3628581184876));
#8481=CARTESIAN_POINT('Ctrl Pts',(0.874893609330296,-0.424537808037555,
10.3973795175289));
#8482=CARTESIAN_POINT('Ctrl Pts',(0.988072988143918,0.0679732521261451,
10.4376022678486));
#8483=CARTESIAN_POINT('Ctrl Pts',(0.792326107474424,0.628891245980529,10.4835024209011));
#8484=CARTESIAN_POINT('Ctrl Pts',(0.226370211101435,0.984231506720089,10.5350532100885));
#8485=CARTESIAN_POINT('Ctrl Pts',(-0.436123968807799,0.909336880303367,
10.5865289946361));
#8486=CARTESIAN_POINT('Ctrl Pts',(-0.907099616963547,0.438321024396503,
10.6379399044686));
#8487=CARTESIAN_POINT('Ctrl Pts',(-0.981413923118005,-0.222912321612607,
10.6892968715003));
#8488=CARTESIAN_POINT('Ctrl Pts',(-0.627778574641029,-0.785671011073721,
10.7406112122533));
#8489=CARTESIAN_POINT('Ctrl Pts',(-0.000441041026566889,-1.00521891170418,
10.7918931531218));
#8490=CARTESIAN_POINT('Ctrl Pts',(0.52144028745575,-0.822006313423052,10.8346123836516));
#8491=CARTESIAN_POINT('Ctrl Pts',(0.803284290233143,-0.504957992571902,
10.8687804323078));
#8492=CARTESIAN_POINT('Ctrl Pts',(0.966617256853383,-0.113399258972559,
10.9029470303529));
#8493=CARTESIAN_POINT('Ctrl Pts',(0.905970307108542,0.43601079523538,10.9456579859439));
#8494=CARTESIAN_POINT('Ctrl Pts',(0.435368363134417,0.906210162272629,10.9969260175495));
#8495=CARTESIAN_POINT('Ctrl Pts',(-0.150964337688312,0.971610417839796,
11.0425194902371));
#8496=CARTESIAN_POINT('Ctrl Pts',(-0.602400284855791,0.753381994777755,
11.0824343495858));
#8497=CARTESIAN_POINT('Ctrl Pts',(-0.870405218502895,0.417758929984093,
11.1166674917653));
#8498=CARTESIAN_POINT('Ctrl Pts',(-0.965973798101014,-0.00153480929624971,
11.1509206149028));
#8499=CARTESIAN_POINT('Ctrl Pts',(-0.870284764404151,-0.421002164664357,
11.1852011748759));
#8500=CARTESIAN_POINT('Ctrl Pts',(-0.601830888141152,-0.757731064011876,
11.2195098193561));
#8501=CARTESIAN_POINT('Ctrl Pts',(-0.213486681158965,-0.944867152397458,
11.2538513120739));
#8502=CARTESIAN_POINT('Ctrl Pts',(0.217961288027539,-0.9447880279063,11.2882255611698));
#8503=CARTESIAN_POINT('Ctrl Pts',(0.607187071933093,-0.757413281709361,
11.3226393123278));
#8504=CARTESIAN_POINT('Ctrl Pts',(0.876844610743522,-0.419393441672649,
11.3570938790573));
#8505=CARTESIAN_POINT('Ctrl Pts',(0.973349361765023,0.00288962313001501,
11.3915922816714));
#8506=CARTESIAN_POINT('Ctrl Pts',(0.876757888575241,0.425354250291934,11.4261375530626));
#8507=CARTESIAN_POINT('Ctrl Pts',(0.561431004887934,0.822273741287479,11.4664977820191));
#8508=CARTESIAN_POINT('Ctrl Pts',(-0.0029686874240922,1.02071711991479,
11.5127131391255));
#8509=CARTESIAN_POINT('Ctrl Pts',(-0.64073387394736,0.797757518731472,11.5648313598225));
#8510=CARTESIAN_POINT('Ctrl Pts',(-1.00104023104205,0.224805257101963,11.6170855603212));
#8511=CARTESIAN_POINT('Ctrl Pts',(-0.925442327878976,-0.449927244069821,
11.6694834791769));
#8512=CARTESIAN_POINT('Ctrl Pts',(-0.444252973113854,-0.931505251605332,
11.7220333653095));
#8513=CARTESIAN_POINT('Ctrl Pts',(0.234224731061071,-1.00859451570503,11.7747423231968));
#8514=CARTESIAN_POINT('Ctrl Pts',(0.81445437030024,-0.644038197480611,11.827617902194));
#8515=CARTESIAN_POINT('Ctrl Pts',(0.965855550860405,-0.212574361888019,
11.8629834282669));
#8516=CARTESIAN_POINT('Ctrl Pts',(0.96588488284949,0.00483552499042606,
11.8806927284981));
#8517=CARTESIAN_POINT('Ctrl Pts',(1.06707985315926,-0.00123476537768325,
8.87526981796726));
#8518=CARTESIAN_POINT('Ctrl Pts',(1.06704748827009,0.238654817693568,8.89481022010543));
#8519=CARTESIAN_POINT('Ctrl Pts',(0.8998395871503,0.715860547817637,8.93391958700505));
#8520=CARTESIAN_POINT('Ctrl Pts',(0.257138893203379,1.11993605733771,8.99249828235584));
#8521=CARTESIAN_POINT('Ctrl Pts',(-0.496179770892746,1.03467055578583,9.05102018674564));
#8522=CARTESIAN_POINT('Ctrl Pts',(-1.03136334290367,0.499226173485843,9.10945853061635));
#8523=CARTESIAN_POINT('Ctrl Pts',(-1.11588620841635,-0.25201787262317,9.16781107428167));
#8524=CARTESIAN_POINT('Ctrl Pts',(-0.713942264474925,-0.890966581948507,
9.22606298427746));
#8525=CARTESIAN_POINT('Ctrl Pts',(-0.21059029264254,-1.06682548550579,9.26725052311974));
#8526=CARTESIAN_POINT('Ctrl Pts',(0.0855976314555819,-1.054052987163,9.29144852924291));
#8527=CARTESIAN_POINT('Ctrl Pts',(0.203192078226194,-1.03916618931912,9.30112514367417));
#8528=CARTESIAN_POINT('Ctrl Pts',(0.347031573799707,-1.00207044132561,9.31321650524867));
#8529=CARTESIAN_POINT('Ctrl Pts',(0.509545413954052,-0.929248527148037,
9.32771837457598));
#8530=CARTESIAN_POINT('Ctrl Pts',(0.783953494823923,-0.746364639224551,
9.35455933228035));
#8531=CARTESIAN_POINT('Ctrl Pts',(1.06593687748999,-0.332681687964893,9.39370140995972));
#8532=CARTESIAN_POINT('Ctrl Pts',(1.06623597197503,0.325089931912099,9.44506593995741));
#8533=CARTESIAN_POINT('Ctrl Pts',(0.727258506600483,0.821784451489806,9.49204879073065));
#8534=CARTESIAN_POINT('Ctrl Pts',(0.244580458213156,1.05328946139207,9.53467422595177));
#8535=CARTESIAN_POINT('Ctrl Pts',(-0.236010419637293,1.05343265745285,9.57296888983229));
#8536=CARTESIAN_POINT('Ctrl Pts',(-0.668252297750573,0.84494474001119,9.61119194755577));
#8537=CARTESIAN_POINT('Ctrl Pts',(-0.96672974583056,0.47053384886532,9.64934284697546));
#8538=CARTESIAN_POINT('Ctrl Pts',(-1.07306322407242,0.00448821120086209,
9.68741884390622));
#8539=CARTESIAN_POINT('Ctrl Pts',(-0.98443925125814,-0.382945442280808,
9.71908515419177));
#8540=CARTESIAN_POINT('Ctrl Pts',(-0.818466620582291,-0.646608252509767,
9.74437859502403));
#8541=CARTESIAN_POINT('Ctrl Pts',(-0.598557383662294,-0.866842730767591,
9.76964562480785));
#8542=CARTESIAN_POINT('Ctrl Pts',(-0.241936616572021,-1.03858706068224,
9.8011796330524));
#8543=CARTESIAN_POINT('Ctrl Pts',(0.232022932609555,-1.03845317207481,9.83893862551647));
#8544=CARTESIAN_POINT('Ctrl Pts',(0.658205813052732,-0.833156021220092,
9.87661449080378));
#8545=CARTESIAN_POINT('Ctrl Pts',(0.952040531211175,-0.464218655543736,
9.91420589839601));
#8546=CARTESIAN_POINT('Ctrl Pts',(1.06912457221153,0.0459190084133642,9.95587871432431));
#8547=CARTESIAN_POINT('Ctrl Pts',(0.896163985835651,0.604804501827073,10.0015953006467));
#8548=CARTESIAN_POINT('Ctrl Pts',(0.481633120790058,0.935455264202716,10.0430249679984));
#8549=CARTESIAN_POINT('Ctrl Pts',(0.0823590282165599,1.02559253520912,10.0760894895048));
#8550=CARTESIAN_POINT('Ctrl Pts',(-0.325147597322649,0.995783918629276,
10.1091010377242));
#8551=CARTESIAN_POINT('Ctrl Pts',(-0.781419164358984,0.732302037853845,
10.1502641539734));
#8552=CARTESIAN_POINT('Ctrl Pts',(-1.05481197310381,0.164416196982754,10.1994999089072));
#8553=CARTESIAN_POINT('Ctrl Pts',(-0.957579147098405,-0.482838702730343,
10.2506175062341));
#8554=CARTESIAN_POINT('Ctrl Pts',(-0.471923124685282,-0.968373088850138,
10.3035915305234));
#8555=CARTESIAN_POINT('Ctrl Pts',(0.155063724599384,-1.03780443842841,10.3523070394179));
#8556=CARTESIAN_POINT('Ctrl Pts',(0.635656486568682,-0.80540414765001,10.3948019151775));
#8557=CARTESIAN_POINT('Ctrl Pts',(0.919506135055416,-0.448974992668351,
10.431135292655));
#8558=CARTESIAN_POINT('Ctrl Pts',(1.03842188491753,0.0688216676404025,10.4734179726515));
#8559=CARTESIAN_POINT('Ctrl Pts',(0.832773812963301,0.657512741565147,10.5215893003721));
#8560=CARTESIAN_POINT('Ctrl Pts',(0.239794832763951,1.02952139718656,10.5755830086345));
#8561=CARTESIAN_POINT('Ctrl Pts',(-0.45262480578768,0.950973831099203,10.6293794921735));
#8562=CARTESIAN_POINT('Ctrl Pts',(-0.943549992884528,0.459607520916314,
10.6829827001157));
#8563=CARTESIAN_POINT('Ctrl Pts',(-1.0205554561502,-0.228234505928641,10.7363967638958));
#8564=CARTESIAN_POINT('Ctrl Pts',(-0.653411141648812,-0.8119181268805,10.7896259939305));
#8565=CARTESIAN_POINT('Ctrl Pts',(-0.00424388176717446,-1.0387549035362,
10.842676676515));
#8566=CARTESIAN_POINT('Ctrl Pts',(0.534047985812385,-0.849488279944819,
10.8867394772746));
#8567=CARTESIAN_POINT('Ctrl Pts',(0.824125963852387,-0.523093463830685,
10.9219091864479));
#8568=CARTESIAN_POINT('Ctrl Pts',(0.991956861439558,-0.120598140671722,
10.9570246594903));
#8569=CARTESIAN_POINT('Ctrl Pts',(0.929487999659989,0.442783713789643,11.0008170365044));
#8570=CARTESIAN_POINT('Ctrl Pts',(0.448174079732207,0.923135490503192,11.0532130656101));
#8571=CARTESIAN_POINT('Ctrl Pts',(-0.149246274677376,0.989455764861352,
11.099658036704));
#8572=CARTESIAN_POINT('Ctrl Pts',(-0.607887737979885,0.767591199020883,
11.1402120021755));
#8573=CARTESIAN_POINT('Ctrl Pts',(-0.879518432239106,0.427263871776012,
11.174912490265));
#8574=CARTESIAN_POINT('Ctrl Pts',(-0.976082172216738,0.00308668187306984,
11.2095606056502));
#8575=CARTESIAN_POINT('Ctrl Pts',(-0.879406973557938,-0.420236621178114,
11.2441531370345));
#8576=CARTESIAN_POINT('Ctrl Pts',(-0.608997527935039,-0.759237523513902,
11.2786964846213));
#8577=CARTESIAN_POINT('Ctrl Pts',(-0.218810131166539,-0.947139071472111,
11.3131910809694));
#8578=CARTESIAN_POINT('Ctrl Pts',(0.213658136544478,-0.94694361480508,11.3476445942225));
#8579=CARTESIAN_POINT('Ctrl Pts',(0.602841583902335,-0.759465040168191,
11.3820544328846));
#8580=CARTESIAN_POINT('Ctrl Pts',(0.871796157798383,-0.422143654068603,
11.4164262050128));
#8581=CARTESIAN_POINT('Ctrl Pts',(0.967743919091153,-0.0017645367439769,
11.4507628656491));
#8582=CARTESIAN_POINT('Ctrl Pts',(0.87170737632655,0.417779623846008,11.4850673080446));
#8583=CARTESIAN_POINT('Ctrl Pts',(0.559133149320638,0.811009041168935,11.5250561770006));
#8584=CARTESIAN_POINT('Ctrl Pts',(0.00135353631370101,1.00676598110684,
11.5707114011782));
#8585=CARTESIAN_POINT('Ctrl Pts',(-0.626564919774301,0.786837182071727,
11.6220280050714));
#8586=CARTESIAN_POINT('Ctrl Pts',(-0.97989246930752,0.224284866953415,11.6733084179627));
#8587=CARTESIAN_POINT('Ctrl Pts',(-0.905576830269774,-0.435795198091819,
11.7245632840688));
#8588=CARTESIAN_POINT('Ctrl Pts',(-0.436058105615478,-0.905191005915266,
11.7758062366315));
#8589=CARTESIAN_POINT('Ctrl Pts',(0.223607192099306,-0.979837529970289,
11.8270420788981));
#8590=CARTESIAN_POINT('Ctrl Pts',(0.785864651600639,-0.626123961781889,
11.8782964306891));
#8591=CARTESIAN_POINT('Ctrl Pts',(0.931965422655655,-0.209149242308135,
11.9124623274458));
#8592=CARTESIAN_POINT('Ctrl Pts',(0.931993756029,0.000858864397959647,11.9295687096166));
#8593=CARTESIAN_POINT('Ctrl Pts',(1.05361350283538,0.00348296873761165,
8.81732980737331));
#8594=CARTESIAN_POINT('Ctrl Pts',(1.0535815233416,0.24051598896115,8.836637525849));
#8595=CARTESIAN_POINT('Ctrl Pts',(0.888483313940475,0.712467681174716,8.8753039923388));
#8596=CARTESIAN_POINT('Ctrl Pts',(0.251129926275458,1.11367978850147,8.93341429944556));
#8597=CARTESIAN_POINT('Ctrl Pts',(-0.498485108509924,1.0291918195949,8.99163796243809));
#8598=CARTESIAN_POINT('Ctrl Pts',(-1.03291163235678,0.495047846251041,9.04996025164164));
#8599=CARTESIAN_POINT('Ctrl Pts',(-1.11791454965682,-0.257013855216408,
9.10837309877508));
#8600=CARTESIAN_POINT('Ctrl Pts',(-0.714602934220277,-0.898858458114211,
9.16686610473355));
#8601=CARTESIAN_POINT('Ctrl Pts',(-0.207691595850096,-1.07623821818795,
9.20834669901183));
#8602=CARTESIAN_POINT('Ctrl Pts',(0.0911678852700241,-1.06335197381873,
9.23276211443464));
#8603=CARTESIAN_POINT('Ctrl Pts',(0.209866246985131,-1.04832623169789,9.24252954635982));
#8604=CARTESIAN_POINT('Ctrl Pts',(0.355138049245429,-1.01086646870226,9.25474086067091));
#8605=CARTESIAN_POINT('Ctrl Pts',(0.519396104990609,-0.937268700996166,
9.26939783627726));
#8606=CARTESIAN_POINT('Ctrl Pts',(0.796954605660454,-0.752300466043746,
9.29654620334218));
#8607=CARTESIAN_POINT('Ctrl Pts',(1.08280563220712,-0.333290926636967,9.3361995653769));
#8608=CARTESIAN_POINT('Ctrl Pts',(1.08337830847036,0.334912126982432,9.38837847049749));
#8609=CARTESIAN_POINT('Ctrl Pts',(0.738315461087922,0.840931330660767,9.43622874255615));
#8610=CARTESIAN_POINT('Ctrl Pts',(0.245636643115447,1.07736261426428,9.47973966869423));
#8611=CARTESIAN_POINT('Ctrl Pts',(-0.245887374235519,1.07760739558264,9.51890418887534));
#8612=CARTESIAN_POINT('Ctrl Pts',(-0.688848319885635,0.864061693882516,
9.55807043542996));
#8613=CARTESIAN_POINT('Ctrl Pts',(-0.995336775626925,0.479757650920096,
9.59723465260094));
#8614=CARTESIAN_POINT('Ctrl Pts',(-1.10479102070153,0.000469460247281091,
9.63639363908221));
#8615=CARTESIAN_POINT('Ctrl Pts',(-1.01355573715264,-0.398724027650001,
9.66901900999136));
#8616=CARTESIAN_POINT('Ctrl Pts',(-0.842337462850113,-0.670747199386004,
9.69511336499282));
#8617=CARTESIAN_POINT('Ctrl Pts',(-0.615278718012576,-0.898162572142696,
9.72120320245627));
#8618=CARTESIAN_POINT('Ctrl Pts',(-0.246601093264737,-1.07579559008464,
9.75380618018306));
#8619=CARTESIAN_POINT('Ctrl Pts',(0.244252856073734,-1.07574552507989,9.79291120095988));
#8620=CARTESIAN_POINT('Ctrl Pts',(0.686391851322618,-0.86285853975462,9.83199461216117));
#8621=CARTESIAN_POINT('Ctrl Pts',(0.991754530098738,-0.479576560375196,
9.87105294828468));
#8622=CARTESIAN_POINT('Ctrl Pts',(1.11368561614542,0.0512633874947476,9.91442019466662));
#8623=CARTESIAN_POINT('Ctrl Pts',(0.933546075553114,0.633941769683682,9.96207896521016));
#8624=CARTESIAN_POINT('Ctrl Pts',(0.500670512163495,0.979417458553777,10.0053529017601));
#8625=CARTESIAN_POINT('Ctrl Pts',(0.0830568987247602,1.07372340050911,10.0399368296195));
#8626=CARTESIAN_POINT('Ctrl Pts',(-0.34353856408149,1.04254504990199,10.0744958406771));
#8627=CARTESIAN_POINT('Ctrl Pts',(-0.821892667873493,0.766467885156324,
10.1176479867357));
#8628=CARTESIAN_POINT('Ctrl Pts',(-1.10907816859822,0.170284170765609,10.1693443469628));
#8629=CARTESIAN_POINT('Ctrl Pts',(-1.00698193012689,-0.510368802257205,
10.2231009495772));
#8630=CARTESIAN_POINT('Ctrl Pts',(-0.495623852462474,-1.02186283833792,
10.2788969581773));
#8631=CARTESIAN_POINT('Ctrl Pts',(0.165675816180989,-1.09524360987832,10.3302841789608));
#8632=CARTESIAN_POINT('Ctrl Pts',(0.673146867597226,-0.849907619411545,
10.3751549170633));
#8633=CARTESIAN_POINT('Ctrl Pts',(0.973126940522068,-0.473284873083087,
10.4135506217634));
#8634=CARTESIAN_POINT('Ctrl Pts',(1.0989251921748,0.0742805190588762,10.4582680283262));
#8635=CARTESIAN_POINT('Ctrl Pts',(0.881352975646305,0.697400663319528,10.5092599474022));
#8636=CARTESIAN_POINT('Ctrl Pts',(0.253250795230376,1.09155624924297,10.5664618213278));
#8637=CARTESIAN_POINT('Ctrl Pts',(-0.48074740256993,1.00836583230992,10.6234942829921));
#8638=CARTESIAN_POINT('Ctrl Pts',(-1.00144411702416,0.487271213800995,10.6803508700943));
#8639=CARTESIAN_POINT('Ctrl Pts',(-1.0831682514647,-0.242479183935224,10.7370260948775));
#8640=CARTESIAN_POINT('Ctrl Pts',(-0.693589794262895,-0.861829276622573,
10.7935153200748));
#8641=CARTESIAN_POINT('Ctrl Pts',(-0.00476094955930445,-1.10250820840403,
10.8498132155155));
#8642=CARTESIAN_POINT('Ctrl Pts',(0.566304342976761,-0.901685114817027,
10.8965673946933));
#8643=CARTESIAN_POINT('Ctrl Pts',(0.873933911656398,-0.55552423775986,10.9338691274573));
#8644=CARTESIAN_POINT('Ctrl Pts',(1.05187813310911,-0.128755879899797,10.9711041860801));
#8645=CARTESIAN_POINT('Ctrl Pts',(0.985595273517537,0.468350561132292,11.0175242489621));
#8646=CARTESIAN_POINT('Ctrl Pts',(0.475749928532382,0.977025441719225,11.0730273616305));
#8647=CARTESIAN_POINT('Ctrl Pts',(-0.156414893216963,1.04708636726262,11.1221822254832));
#8648=CARTESIAN_POINT('Ctrl Pts',(-0.641231356480644,0.812507364268063,
11.1650570351354));
#8649=CARTESIAN_POINT('Ctrl Pts',(-0.928115411763875,0.452991280889662,
11.2017171506232));
#8650=CARTESIAN_POINT('Ctrl Pts',(-1.02997376320952,0.00534914585065388,
11.2382833095929));
#8651=CARTESIAN_POINT('Ctrl Pts',(-0.927988165491989,-0.440956849896211,
11.2747605777941));
#8652=CARTESIAN_POINT('Ctrl Pts',(-0.643147665450665,-0.797961485702993,
11.3111461991335));
#8653=CARTESIAN_POINT('Ctrl Pts',(-0.232622271758171,-0.995586956799243,
11.3474425164299));
#8654=CARTESIAN_POINT('Ctrl Pts',(0.221782139701691,-0.995323011688169,
11.3836461234341));
#8655=CARTESIAN_POINT('Ctrl Pts',(0.630176503673988,-0.798514686074851,
11.4197621600222));
#8656=CARTESIAN_POINT('Ctrl Pts',(0.911993998160867,-0.444953718020728,
11.4557892580011));
#8657=CARTESIAN_POINT('Ctrl Pts',(1.0123375157838,-0.00499677880190555,
11.4917283504049));
#8658=CARTESIAN_POINT('Ctrl Pts',(0.911913781362388,0.433400322908333,11.5275805946167));
#8659=CARTESIAN_POINT('Ctrl Pts',(0.585711603391555,0.843623662983355,11.5693073793534));
#8660=CARTESIAN_POINT('Ctrl Pts',(0.00481853796942386,1.04723189572395,
11.6168567678419));
#8661=CARTESIAN_POINT('Ctrl Pts',(-0.647234763521536,0.818520165995884,
11.6701623256145));
#8662=CARTESIAN_POINT('Ctrl Pts',(-1.01294419891713,0.2356558517606,11.7232877007132));
#8663=CARTESIAN_POINT('Ctrl Pts',(-0.935844923634562,-0.446106838298428,
11.7762368087852));
#8664=CARTESIAN_POINT('Ctrl Pts',(-0.452045047065324,-0.929290107925388,
11.8290183926509));
#8665=CARTESIAN_POINT('Ctrl Pts',(0.225347069308191,-1.00558585215721,11.8816338257412));
#8666=CARTESIAN_POINT('Ctrl Pts',(0.800671735601205,-0.643237553051006,
11.9341015844704));
#8667=CARTESIAN_POINT('Ctrl Pts',(0.949567997660912,-0.217730099299315,
11.9689677728214));
#8668=CARTESIAN_POINT('Ctrl Pts',(0.949596863894161,-0.00377241348101253,
11.9863958711905));
#8669=CARTESIAN_POINT('Ctrl Pts',(1.01795130065334,0.00487363731203012,
8.80019806641107));
#8670=CARTESIAN_POINT('Ctrl Pts',(1.01792038659565,0.234009611419109,8.81886252453821));
#8671=CARTESIAN_POINT('Ctrl Pts',(0.858367966757573,0.690235048013234,8.85624002408532));
#8672=CARTESIAN_POINT('Ctrl Pts',(0.241569528156157,1.07870571562318,8.91248661418056));
#8673=CARTESIAN_POINT('Ctrl Pts',(-0.484837290617098,0.996972530018084,
8.96890545081248));
#8674=CARTESIAN_POINT('Ctrl Pts',(-1.00348249888983,0.478852252916471,9.02549359964913));
#8675=CARTESIAN_POINT('Ctrl Pts',(-1.08625117261773,-0.25179645236032,9.08224516844789));
#8676=CARTESIAN_POINT('Ctrl Pts',(-0.694018194752758,-0.876373474596457,
9.13915599966505));
#8677=CARTESIAN_POINT('Ctrl Pts',(-0.200132218465017,-1.04934671836633,
9.17957488341133));
#8678=CARTESIAN_POINT('Ctrl Pts',(0.0913368318045304,-1.03678149851834,
9.20338638692998));
#8679=CARTESIAN_POINT('Ctrl Pts',(0.207121875172981,-1.02212501822983,9.21291409202708));
#8680=CARTESIAN_POINT('Ctrl Pts',(0.348871161210955,-0.985577072042873,
9.22482919048418));
#8681=CARTESIAN_POINT('Ctrl Pts',(0.509211865524956,-0.913738037165839,
9.23913636256541));
#8682=CARTESIAN_POINT('Ctrl Pts',(0.780259255512014,-0.733117828399737,
9.26564749781129));
#8683=CARTESIAN_POINT('Ctrl Pts',(1.05975444985038,-0.323629573613465,9.30440431224551));
#8684=CARTESIAN_POINT('Ctrl Pts',(1.06047114568476,0.330478386785373,9.3554821017605));
#8685=CARTESIAN_POINT('Ctrl Pts',(0.722286003799723,0.826672635352907,9.40239348796624));
#8686=CARTESIAN_POINT('Ctrl Pts',(0.238614159531519,1.05887024839816,9.44510997373937));
#8687=CARTESIAN_POINT('Ctrl Pts',(-0.244534897444566,1.0591832153207,9.48360493669715));
#8688=CARTESIAN_POINT('Ctrl Pts',(-0.680524248557215,0.849074843118668,
9.52215116753634));
#8689=CARTESIAN_POINT('Ctrl Pts',(-0.98259760908771,0.470426970871326,9.56074113449322));
#8690=CARTESIAN_POINT('Ctrl Pts',(-1.09066217491685,-0.00244906966523479,
9.59937538820734));
#8691=CARTESIAN_POINT('Ctrl Pts',(-1.00058931413245,-0.396830955934259,
9.63160353230798));
#8692=CARTESIAN_POINT('Ctrl Pts',(-0.831280757584498,-0.66584407874337,
9.65740738981046));
#8693=CARTESIAN_POINT('Ctrl Pts',(-0.60660620885125,-0.890890186335246,
9.68322356907152));
#8694=CARTESIAN_POINT('Ctrl Pts',(-0.241464397156938,-1.06689249054125,
9.71551297140233));
#8695=CARTESIAN_POINT('Ctrl Pts',(0.245368155864266,-1.06692104952396,9.75429461177334));
#8696=CARTESIAN_POINT('Ctrl Pts',(0.684501955300456,-0.855569813249952,
9.79310524648812));
#8697=CARTESIAN_POINT('Ctrl Pts',(0.988229478846218,-0.474457482452504,
9.83194393027524));
#8698=CARTESIAN_POINT('Ctrl Pts',(1.10973816459222,0.0541175025352953,9.87512290940774));
#8699=CARTESIAN_POINT('Ctrl Pts',(0.930219960144453,0.635314767499316,9.92265302971509));
#8700=CARTESIAN_POINT('Ctrl Pts',(0.497804230880996,0.980626921647988,9.96588699941796));
#8701=CARTESIAN_POINT('Ctrl Pts',(0.0799630716897277,1.07501359287928,10.0004861839901));
#8702=CARTESIAN_POINT('Ctrl Pts',(-0.347252228161148,1.04382229510122,10.0350937644591));
#8703=CARTESIAN_POINT('Ctrl Pts',(-0.826997276535407,0.767113462252174,
10.0783561346641));
#8704=CARTESIAN_POINT('Ctrl Pts',(-1.11568341591399,0.168249508212943,10.1302891091875));
#8705=CARTESIAN_POINT('Ctrl Pts',(-1.01311996047222,-0.516807562056236,
10.1843847097011));
#8706=CARTESIAN_POINT('Ctrl Pts',(-0.497693146880373,-1.03272594487734,
10.2406345323798));
#8707=CARTESIAN_POINT('Ctrl Pts',(0.170406057393102,-1.10708621318768,10.2925411425343));
#8708=CARTESIAN_POINT('Ctrl Pts',(0.684033423898933,-0.858869402467361,
10.3379484762471));
#8709=CARTESIAN_POINT('Ctrl Pts',(0.988073809172079,-0.477253180864907,
10.3768544364604));
#8710=CARTESIAN_POINT('Ctrl Pts',(1.11580410768175,0.0783050484260798,10.4222217990858));
#8711=CARTESIAN_POINT('Ctrl Pts',(0.89490232388525,0.711594886645981,10.4740302655834));
#8712=CARTESIAN_POINT('Ctrl Pts',(0.255533065555895,1.11310545631092,10.5322604116042));
#8713=CARTESIAN_POINT('Ctrl Pts',(-0.493177190634868,1.028473309878,10.5904230992472));
#8714=CARTESIAN_POINT('Ctrl Pts',(-1.02539476057429,0.496166178496065,10.6485098680401));
#8715=CARTESIAN_POINT('Ctrl Pts',(-1.10926310066815,-0.250769149465673,
10.7065110803908));
#8716=CARTESIAN_POINT('Ctrl Pts',(-0.710019491092949,-0.885888782146993,
10.7644169839348));
#8717=CARTESIAN_POINT('Ctrl Pts',(-0.00271517191512337,-1.13323556057773,
10.8222205409864));
#8718=CARTESIAN_POINT('Ctrl Pts',(0.584651230956468,-0.926841543599498,
10.8702938955112));
#8719=CARTESIAN_POINT('Ctrl Pts',(0.901430071020036,-0.570430111687275,
10.9086978561871));
#8720=CARTESIAN_POINT('Ctrl Pts',(1.08480128691465,-0.130713242941942,10.9470608547078));
#8721=CARTESIAN_POINT('Ctrl Pts',(1.01658557007516,0.485161030998729,10.9949317431856));
#8722=CARTESIAN_POINT('Ctrl Pts',(0.490173403409379,1.01059242800624,11.0522381720562));
#8723=CARTESIAN_POINT('Ctrl Pts',(-0.163448336991982,1.08316288382942,11.103050538961));
#8724=CARTESIAN_POINT('Ctrl Pts',(-0.665244137705534,0.840414645124265,
11.1474196034443));
#8725=CARTESIAN_POINT('Ctrl Pts',(-0.962390571076912,0.468100768895086,
11.1853798655439));
#8726=CARTESIAN_POINT('Ctrl Pts',(-1.06798711473851,0.00416599671308398,
11.2232748034332));
#8727=CARTESIAN_POINT('Ctrl Pts',(-0.962266470067073,-0.458657680157008,
11.2610950285115));
#8728=CARTESIAN_POINT('Ctrl Pts',(-0.666738558731371,-0.829099316917844,
11.2988435852598));
#8729=CARTESIAN_POINT('Ctrl Pts',(-0.240581161310417,-1.03428058472939,
11.3365161841455));
#8730=CARTESIAN_POINT('Ctrl Pts',(0.23139593208825,-1.03402414691513,11.37411710958));
#8731=CARTESIAN_POINT('Ctrl Pts',(0.655753330921873,-0.829545509919698,
11.4116386576741));
#8732=CARTESIAN_POINT('Ctrl Pts',(0.948704829357944,-0.462037948503457,
11.4490826297383));
#8733=CARTESIAN_POINT('Ctrl Pts',(1.05305294362534,-0.00456577157253448,
11.4864478733918));
#8734=CARTESIAN_POINT('Ctrl Pts',(0.948608126586202,0.451416711858766,11.523733236039));
#8735=CARTESIAN_POINT('Ctrl Pts',(0.609246817799872,0.878201568608402,11.5671395812719));
#8736=CARTESIAN_POINT('Ctrl Pts',(0.00480141380439488,1.09007650729612,
11.6166080030503));
#8737=CARTESIAN_POINT('Ctrl Pts',(-0.673807025591558,0.852056511070549,
11.6720765353948));
#8738=CARTESIAN_POINT('Ctrl Pts',(-1.05440803560707,0.245435452705016,11.7273583516172));
#8739=CARTESIAN_POINT('Ctrl Pts',(-0.974155187242797,-0.464027523123006,
11.7824525288063));
#8740=CARTESIAN_POINT('Ctrl Pts',(-0.470784479502001,-0.966711922017756,
11.837360017147));
#8741=CARTESIAN_POINT('Ctrl Pts',(0.233728487300451,-1.0459922691019,11.8920770765874));
#8742=CARTESIAN_POINT('Ctrl Pts',(0.831757325146403,-0.66927695668899,11.9466131794695));
#8743=CARTESIAN_POINT('Ctrl Pts',(0.986370555206023,-0.227123217897721,
11.9828356523871));
#8744=CARTESIAN_POINT('Ctrl Pts',(0.986400528300369,-0.00496143295807807,
12.0009320223632));
#8745=CARTESIAN_POINT('Ctrl Pts',(0.999999342796208,0.0048712153097108,
8.80019806641107));
#8746=CARTESIAN_POINT('Ctrl Pts',(0.99996896462742,0.230035163961994,8.81853897995701));
#8747=CARTESIAN_POINT('Ctrl Pts',(0.843216945008081,0.678245689353448,8.85526000727444));
#8748=CARTESIAN_POINT('Ctrl Pts',(0.23714388778331,1.05999084182087,8.91053070559157));
#8749=CARTESIAN_POINT('Ctrl Pts',(-0.476746387578999,0.979670338171269,
8.96597705173729));
#8750=CARTESIAN_POINT('Ctrl Pts',(-0.98657616663209,0.470389879273211,9.0216024298575));
#8751=CARTESIAN_POINT('Ctrl Pts',(-1.06798165663575,-0.248000588468906,
9.07740270249169));
#8752=CARTESIAN_POINT('Ctrl Pts',(-0.682243081073035,-0.862304425765768,
9.1333764236107));
#8753=CARTESIAN_POINT('Ctrl Pts',(-0.196330490445415,-1.03251494397982,
9.17314484390509));
#8754=CARTESIAN_POINT('Ctrl Pts',(0.0904960552365201,-1.02015022040365,
9.19657718102618));
#8755=CARTESIAN_POINT('Ctrl Pts',(0.204441911777542,-1.00572651008441,9.20595357869542));
#8756=CARTESIAN_POINT('Ctrl Pts',(0.343951015893895,-0.96975630344906,9.21768054548145));
#8757=CARTESIAN_POINT('Ctrl Pts',(0.501773879908335,-0.899045416054097,
9.23176320323934));
#8758=CARTESIAN_POINT('Ctrl Pts',(0.768592409823833,-0.721243151610969,
9.2578611494339));
#8759=CARTESIAN_POINT('Ctrl Pts',(1.04382114359922,-0.318042243912805,9.29602676229045));
#8760=CARTESIAN_POINT('Ctrl Pts',(1.04456490155922,0.326294295864951,9.34634267499162));
#8761=CARTESIAN_POINT('Ctrl Pts',(0.711307557250243,0.815326125223123,9.39257751006242));
#8762=CARTESIAN_POINT('Ctrl Pts',(0.234442425347365,1.04427973165066,9.43469552996756));
#8763=CARTESIAN_POINT('Ctrl Pts',(-0.242097506080382,1.04460426316974,9.47266669612882));
#8764=CARTESIAN_POINT('Ctrl Pts',(-0.672296189994615,0.837312084419627,
9.51070107270169));
#8765=CARTESIAN_POINT('Ctrl Pts',(-0.970493141256397,0.463551157181226,
9.54879683116503));
#8766=CARTESIAN_POINT('Ctrl Pts',(-1.07723336834064,-0.00342794058422688,
9.58695206272228));
#8767=CARTESIAN_POINT('Ctrl Pts',(-0.988260429843343,-0.39307851175747,
9.61879599421848));
#8768=CARTESIAN_POINT('Ctrl Pts',(-0.82093539560644,-0.658946730224756,
9.64429884892662));
#8769=CARTESIAN_POINT('Ctrl Pts',(-0.598840710302034,-0.88141322392247,
9.66981982299092));
#8770=CARTESIAN_POINT('Ctrl Pts',(-0.237756057923814,-1.05547919442497,
9.70175433946707));
#8771=CARTESIAN_POINT('Ctrl Pts',(0.243905786180905,-1.05553040152794,9.74012683420727));
#8772=CARTESIAN_POINT('Ctrl Pts',(0.678604028637572,-0.846341399380819,
9.77854812145871));
#8773=CARTESIAN_POINT('Ctrl Pts',(0.979430107833126,-0.468912235308927,
9.81701586224876));
#8774=CARTESIAN_POINT('Ctrl Pts',(1.09985901046267,0.0548445677701001,9.85980673545165));
#8775=CARTESIAN_POINT('Ctrl Pts',(0.921933505746503,0.631124795915794,9.90693599171239));
#8776=CARTESIAN_POINT('Ctrl Pts',(0.4929126040201,0.973793160670524,9.94983738646297));
#8777=CARTESIAN_POINT('Ctrl Pts',(0.0780904371091028,1.06751269479759,9.98418939216924));
#8778=CARTESIAN_POINT('Ctrl Pts',(-0.346188348797786,1.0365452542535,10.0185609429505));
#8779=CARTESIAN_POINT('Ctrl Pts',(-0.822968443953264,0.76162232341949,10.0615600576428));
#8780=CARTESIAN_POINT('Ctrl Pts',(-1.11011929233597,0.166104281872854,10.1132080400722));
#8781=CARTESIAN_POINT('Ctrl Pts',(-1.0081246602054,-0.515708350877839,10.1670522944212));
#8782=CARTESIAN_POINT('Ctrl Pts',(-0.494775946618556,-1.02970801548153,
10.2230915794475));
#8783=CARTESIAN_POINT('Ctrl Pts',(0.171330015334639,-1.10394798748412,10.2748519542969));
#8784=CARTESIAN_POINT('Ctrl Pts',(0.683814393710209,-0.85633240678914,10.3201591760856));
#8785=CARTESIAN_POINT('Ctrl Pts',(0.987375224349673,-0.475369257557772,
10.3590026286433));
#8786=CARTESIAN_POINT('Ctrl Pts',(1.11501021817459,0.0796008030233853,10.4043267361272));
#8787=CARTESIAN_POINT('Ctrl Pts',(0.894257942603671,0.712772351603783,10.4561304980607));
#8788=CARTESIAN_POINT('Ctrl Pts',(0.254526418580225,1.11465334671006,10.5144063331842));
#8789=CARTESIAN_POINT('Ctrl Pts',(-0.495386650979013,1.03000796421648,10.5726689321936));
#8790=CARTESIAN_POINT('Ctrl Pts',(-1.02902006816757,0.496451864872819,10.6309084916996));
#8791=CARTESIAN_POINT('Ctrl Pts',(-1.11329107431628,-0.25302544687232,10.6891152782939));
#8792=CARTESIAN_POINT('Ctrl Pts',(-0.712411475504087,-0.890954531307481,
10.7472796615617));
#8793=CARTESIAN_POINT('Ctrl Pts',(-0.00144545535703713,-1.13970545531556,
10.8053921361455));
#8794=CARTESIAN_POINT('Ctrl Pts',(0.589562318042014,-0.932130645422847,
10.8537681412278));
#8795=CARTESIAN_POINT('Ctrl Pts',(0.908494555547074,-0.573322783618425,
10.8924337348326));
#8796=CARTESIAN_POINT('Ctrl Pts',(1.0932000203843,-0.130460109720627,10.9310743576345));
#8797=CARTESIAN_POINT('Ctrl Pts',(1.02452819258886,0.49024714203063,10.9793255246093));
#8798=CARTESIAN_POINT('Ctrl Pts',(0.493612168598575,1.02033558321459,11.037138824411));
#8799=CARTESIAN_POINT('Ctrl Pts',(-0.166230575259128,1.09368100121347,11.0884425957329));
#8800=CARTESIAN_POINT('Ctrl Pts',(-0.673140522140151,0.84850197959383,11.1332655331794));
#8801=CARTESIAN_POINT('Ctrl Pts',(-0.973483979429893,0.47222295927322,11.1716363210045));
#8802=CARTESIAN_POINT('Ctrl Pts',(-1.08028898641827,0.00311472479435195,
11.2099559586628));
#8803=CARTESIAN_POINT('Ctrl Pts',(-0.973354083483389,-0.465125791076451,
11.2482222395404));
#8804=CARTESIAN_POINT('Ctrl Pts',(-0.674252322492463,-0.840091585392608,
11.2864330284043));
#8805=CARTESIAN_POINT('Ctrl Pts',(-0.242715089956039,-1.04789098180051,
11.3245862592493));
#8806=CARTESIAN_POINT('Ctrl Pts',(0.23542767696283,-1.04765866302507,11.3626799542613));
#8807=CARTESIAN_POINT('Ctrl Pts',(0.665536159094464,-0.840435751119737,
11.4007121983223));
#8808=CARTESIAN_POINT('Ctrl Pts',(0.962591820228485,-0.467820172164233,
11.4386811727585));
#8809=CARTESIAN_POINT('Ctrl Pts',(1.06846208937938,-0.00379118886353965,
11.47658513569));
#8810=CARTESIAN_POINT('Ctrl Pts',(0.962501175338684,0.458913289962351,11.5144224357756));
#8811=CARTESIAN_POINT('Ctrl Pts',(0.618041205754224,0.892154566858533,11.5584863515166));
#8812=CARTESIAN_POINT('Ctrl Pts',(0.00421838652791971,1.10738146763147,
11.6087289304493));
#8813=CARTESIAN_POINT('Ctrl Pts',(-0.685284502455283,0.86560690604705,11.6650903417562));
#8814=CARTESIAN_POINT('Ctrl Pts',(-1.07219887432344,0.249028474249683,11.7212863124465));
#8815=CARTESIAN_POINT('Ctrl Pts',(-0.990640181337795,-0.472396051339649,
11.7773128627812));
#8816=CARTESIAN_POINT('Ctrl Pts',(-0.478640001005609,-0.983760746265736,
11.8331676524783));
#8817=CARTESIAN_POINT('Ctrl Pts',(0.238202676882345,-1.06445286799178,11.8888462567429));
#8818=CARTESIAN_POINT('Ctrl Pts',(0.846858663881909,-0.681098479204223,
11.9443505326692));
#8819=CARTESIAN_POINT('Ctrl Pts',(1.00427568511571,-0.230977292777482,11.9812290386622));
#8820=CARTESIAN_POINT('Ctrl Pts',(1.00430619197361,-0.004859230773597,11.9996476704237));
#8821=CARTESIAN_POINT('',(0.999999342796208,0.00487121530971084,8.80019806641107));
#8822=CARTESIAN_POINT('Origin',(1.,0.,8.86));
#8823=CARTESIAN_POINT('',(1.00430619197361,-0.00485923077359697,11.9996476704237));
#8824=CARTESIAN_POINT('Ctrl Pts',(0.999999342796208,0.0048712153097108,
8.80019806641107));
#8825=CARTESIAN_POINT('Ctrl Pts',(0.99996896462742,0.230035163961994,8.81853897995701));
#8826=CARTESIAN_POINT('Ctrl Pts',(0.843216945008081,0.678245689353448,8.85526000727444));
#8827=CARTESIAN_POINT('Ctrl Pts',(0.23714388778331,1.05999084182087,8.91053070559157));
#8828=CARTESIAN_POINT('Ctrl Pts',(-0.476746387578999,0.979670338171269,
8.96597705173729));
#8829=CARTESIAN_POINT('Ctrl Pts',(-0.98657616663209,0.470389879273211,9.0216024298575));
#8830=CARTESIAN_POINT('Ctrl Pts',(-1.06798165663575,-0.248000588468906,
9.07740270249169));
#8831=CARTESIAN_POINT('Ctrl Pts',(-0.682243081073035,-0.862304425765768,
9.1333764236107));
#8832=CARTESIAN_POINT('Ctrl Pts',(-0.196330490445415,-1.03251494397982,
9.17314484390509));
#8833=CARTESIAN_POINT('Ctrl Pts',(0.0904960552365201,-1.02015022040365,
9.19657718102618));
#8834=CARTESIAN_POINT('Ctrl Pts',(0.204441911777542,-1.00572651008441,9.20595357869542));
#8835=CARTESIAN_POINT('Ctrl Pts',(0.343951015893895,-0.96975630344906,9.21768054548145));
#8836=CARTESIAN_POINT('Ctrl Pts',(0.501773879908335,-0.899045416054097,
9.23176320323934));
#8837=CARTESIAN_POINT('Ctrl Pts',(0.768592409823833,-0.721243151610969,
9.2578611494339));
#8838=CARTESIAN_POINT('Ctrl Pts',(1.04382114359922,-0.318042243912805,9.29602676229045));
#8839=CARTESIAN_POINT('Ctrl Pts',(1.04456490155922,0.326294295864951,9.34634267499162));
#8840=CARTESIAN_POINT('Ctrl Pts',(0.711307557250243,0.815326125223123,9.39257751006242));
#8841=CARTESIAN_POINT('Ctrl Pts',(0.234442425347365,1.04427973165066,9.43469552996756));
#8842=CARTESIAN_POINT('Ctrl Pts',(-0.242097506080382,1.04460426316974,9.47266669612882));
#8843=CARTESIAN_POINT('Ctrl Pts',(-0.672296189994615,0.837312084419627,
9.51070107270169));
#8844=CARTESIAN_POINT('Ctrl Pts',(-0.970493141256397,0.463551157181226,
9.54879683116503));
#8845=CARTESIAN_POINT('Ctrl Pts',(-1.07723336834064,-0.00342794058422688,
9.58695206272228));
#8846=CARTESIAN_POINT('Ctrl Pts',(-0.988260429843343,-0.39307851175747,
9.61879599421848));
#8847=CARTESIAN_POINT('Ctrl Pts',(-0.82093539560644,-0.658946730224756,
9.64429884892662));
#8848=CARTESIAN_POINT('Ctrl Pts',(-0.598840710302034,-0.88141322392247,
9.66981982299092));
#8849=CARTESIAN_POINT('Ctrl Pts',(-0.237756057923814,-1.05547919442497,
9.70175433946707));
#8850=CARTESIAN_POINT('Ctrl Pts',(0.243905786180905,-1.05553040152794,9.74012683420727));
#8851=CARTESIAN_POINT('Ctrl Pts',(0.678604028637572,-0.846341399380819,
9.77854812145871));
#8852=CARTESIAN_POINT('Ctrl Pts',(0.979430107833126,-0.468912235308927,
9.81701586224876));
#8853=CARTESIAN_POINT('Ctrl Pts',(1.09985901046267,0.0548445677701001,9.85980673545165));
#8854=CARTESIAN_POINT('Ctrl Pts',(0.921933505746503,0.631124795915794,9.90693599171239));
#8855=CARTESIAN_POINT('Ctrl Pts',(0.4929126040201,0.973793160670524,9.94983738646297));
#8856=CARTESIAN_POINT('Ctrl Pts',(0.0780904371091028,1.06751269479759,9.98418939216924));
#8857=CARTESIAN_POINT('Ctrl Pts',(-0.346188348797786,1.0365452542535,10.0185609429505));
#8858=CARTESIAN_POINT('Ctrl Pts',(-0.822968443953264,0.76162232341949,10.0615600576428));
#8859=CARTESIAN_POINT('Ctrl Pts',(-1.11011929233597,0.166104281872854,10.1132080400722));
#8860=CARTESIAN_POINT('Ctrl Pts',(-1.0081246602054,-0.515708350877839,10.1670522944212));
#8861=CARTESIAN_POINT('Ctrl Pts',(-0.494775946618556,-1.02970801548153,
10.2230915794475));
#8862=CARTESIAN_POINT('Ctrl Pts',(0.171330015334639,-1.10394798748412,10.2748519542969));
#8863=CARTESIAN_POINT('Ctrl Pts',(0.683814393710209,-0.85633240678914,10.3201591760856));
#8864=CARTESIAN_POINT('Ctrl Pts',(0.987375224349673,-0.475369257557772,
10.3590026286433));
#8865=CARTESIAN_POINT('Ctrl Pts',(1.11501021817459,0.0796008030233853,10.4043267361272));
#8866=CARTESIAN_POINT('Ctrl Pts',(0.894257942603671,0.712772351603783,10.4561304980607));
#8867=CARTESIAN_POINT('Ctrl Pts',(0.254526418580225,1.11465334671006,10.5144063331842));
#8868=CARTESIAN_POINT('Ctrl Pts',(-0.495386650979013,1.03000796421648,10.5726689321936));
#8869=CARTESIAN_POINT('Ctrl Pts',(-1.02902006816757,0.496451864872819,10.6309084916996));
#8870=CARTESIAN_POINT('Ctrl Pts',(-1.11329107431628,-0.25302544687232,10.6891152782939));
#8871=CARTESIAN_POINT('Ctrl Pts',(-0.712411475504087,-0.890954531307481,
10.7472796615617));
#8872=CARTESIAN_POINT('Ctrl Pts',(-0.00144545535703713,-1.13970545531556,
10.8053921361455));
#8873=CARTESIAN_POINT('Ctrl Pts',(0.589562318042014,-0.932130645422847,
10.8537681412278));
#8874=CARTESIAN_POINT('Ctrl Pts',(0.908494555547074,-0.573322783618425,
10.8924337348326));
#8875=CARTESIAN_POINT('Ctrl Pts',(1.0932000203843,-0.130460109720627,10.9310743576345));
#8876=CARTESIAN_POINT('Ctrl Pts',(1.02452819258886,0.49024714203063,10.9793255246093));
#8877=CARTESIAN_POINT('Ctrl Pts',(0.493612168598575,1.02033558321459,11.037138824411));
#8878=CARTESIAN_POINT('Ctrl Pts',(-0.166230575259128,1.09368100121347,11.0884425957329));
#8879=CARTESIAN_POINT('Ctrl Pts',(-0.673140522140151,0.84850197959383,11.1332655331794));
#8880=CARTESIAN_POINT('Ctrl Pts',(-0.973483979429893,0.47222295927322,11.1716363210045));
#8881=CARTESIAN_POINT('Ctrl Pts',(-1.08028898641827,0.00311472479435195,
11.2099559586628));
#8882=CARTESIAN_POINT('Ctrl Pts',(-0.973354083483389,-0.465125791076451,
11.2482222395404));
#8883=CARTESIAN_POINT('Ctrl Pts',(-0.674252322492463,-0.840091585392608,
11.2864330284043));
#8884=CARTESIAN_POINT('Ctrl Pts',(-0.242715089956039,-1.04789098180051,
11.3245862592493));
#8885=CARTESIAN_POINT('Ctrl Pts',(0.23542767696283,-1.04765866302507,11.3626799542613));
#8886=CARTESIAN_POINT('Ctrl Pts',(0.665536159094464,-0.840435751119737,
11.4007121983223));
#8887=CARTESIAN_POINT('Ctrl Pts',(0.962591820228485,-0.467820172164233,
11.4386811727585));
#8888=CARTESIAN_POINT('Ctrl Pts',(1.06846208937938,-0.00379118886353965,
11.47658513569));
#8889=CARTESIAN_POINT('Ctrl Pts',(0.962501175338684,0.458913289962351,11.5144224357756));
#8890=CARTESIAN_POINT('Ctrl Pts',(0.618041205754224,0.892154566858533,11.5584863515166));
#8891=CARTESIAN_POINT('Ctrl Pts',(0.00421838652791971,1.10738146763147,
11.6087289304493));
#8892=CARTESIAN_POINT('Ctrl Pts',(-0.685284502455283,0.86560690604705,11.6650903417562));
#8893=CARTESIAN_POINT('Ctrl Pts',(-1.07219887432344,0.249028474249683,11.7212863124465));
#8894=CARTESIAN_POINT('Ctrl Pts',(-0.990640181337795,-0.472396051339649,
11.7773128627812));
#8895=CARTESIAN_POINT('Ctrl Pts',(-0.478640001005609,-0.983760746265736,
11.8331676524783));
#8896=CARTESIAN_POINT('Ctrl Pts',(0.238202676882345,-1.06445286799178,11.8888462567429));
#8897=CARTESIAN_POINT('Ctrl Pts',(0.846858663881909,-0.681098479204223,
11.9443505326692));
#8898=CARTESIAN_POINT('Ctrl Pts',(1.00427568511571,-0.230977292777482,11.9812290386622));
#8899=CARTESIAN_POINT('Ctrl Pts',(1.00430619197361,-0.004859230773597,11.9996476704237));
#8900=CARTESIAN_POINT('Origin',(1.,-1.33226762955019E-15,11.94));
#8901=CARTESIAN_POINT('Origin',(1.,-1.33226762955019E-15,11.94));
#8902=CARTESIAN_POINT('Origin',(1.,0.,8.86));
#10198=UNCERTAINTY_MEASURE_WITH_UNIT(LENGTH_MEASURE(0.001),#10266,
'DISTANCE_ACCURACY_VALUE',
'Maximum model space distance between geometric entities at asserted c
onnectivities');
#10227=UNCERTAINTY_MEASURE_WITH_UNIT(LENGTH_MEASURE(0.001),#10266,
'DISTANCE_ACCURACY_VALUE',
'Maximum model space distance between geometric entities at asserted c
onnectivities');
#10236=(
GEOMETRIC_REPRESENTATION_CONTEXT(3)
GLOBAL_UNCERTAINTY_ASSIGNED_CONTEXT((#10198))
GLOBAL_UNIT_ASSIGNED_CONTEXT((#10266,#10268,#10269))
REPRESENTATION_CONTEXT('','3D')
);
#10265=(
GEOMETRIC_REPRESENTATION_CONTEXT(3)
GLOBAL_UNCERTAINTY_ASSIGNED_CONTEXT((#10227))
GLOBAL_UNIT_ASSIGNED_CONTEXT((#10266,#10268,#10269))
REPRESENTATION_CONTEXT('','3D')
);
#10266=(
LENGTH_UNIT()
NAMED_UNIT(*)
SI_UNIT(.CENTI.,.METRE.)
);
#10268=(
NAMED_UNIT(*)
PLANE_ANGLE_UNIT()
SI_UNIT($,.RADIAN.)
);
#10269=(
NAMED_UNIT(*)
SI_UNIT($,.STERADIAN.)
SOLID_ANGLE_UNIT()
);
#10278=SHAPE_DEFINITION_REPRESENTATION(#10315,#10412);
#10315=PRODUCT_DEFINITION_SHAPE('',$,#10450);
#10412=SHAPE_REPRESENTATION('',(#5578),#10236);
#10441=PRODUCT_DEFINITION_CONTEXT('part definition',#10554,'design');
#10450=PRODUCT_DEFINITION('Installed return spring',
'Installed return spring',#10487,#10441);
#10487=PRODUCT_DEFINITION_FORMATION('',$,#10564);
#10554=APPLICATION_CONTEXT(
'Core Data for Automotive Mechanical Design Process');
#10555=PRODUCT_CONTEXT('part definition',#10554,'mechanical');
#10564=PRODUCT('Installed return spring','Installed return spring',
'Installed return spring',(#10555));
#10649=COLOUR_RGB('Grey',0.48,0.52,0.57);
#10650=FILL_AREA_STYLE_COLOUR('',#10649);
#10651=FILL_AREA_STYLE('',(#10650));
#10652=SURFACE_STYLE_FILL_AREA(#10651);
#10653=SURFACE_SIDE_STYLE('',(#10652));
#10654=SURFACE_STYLE_USAGE(.BOTH.,#10653);
#10655=PRESENTATION_STYLE_ASSIGNMENT((#10654));
ENDSEC;
END-ISO-10303-21;
